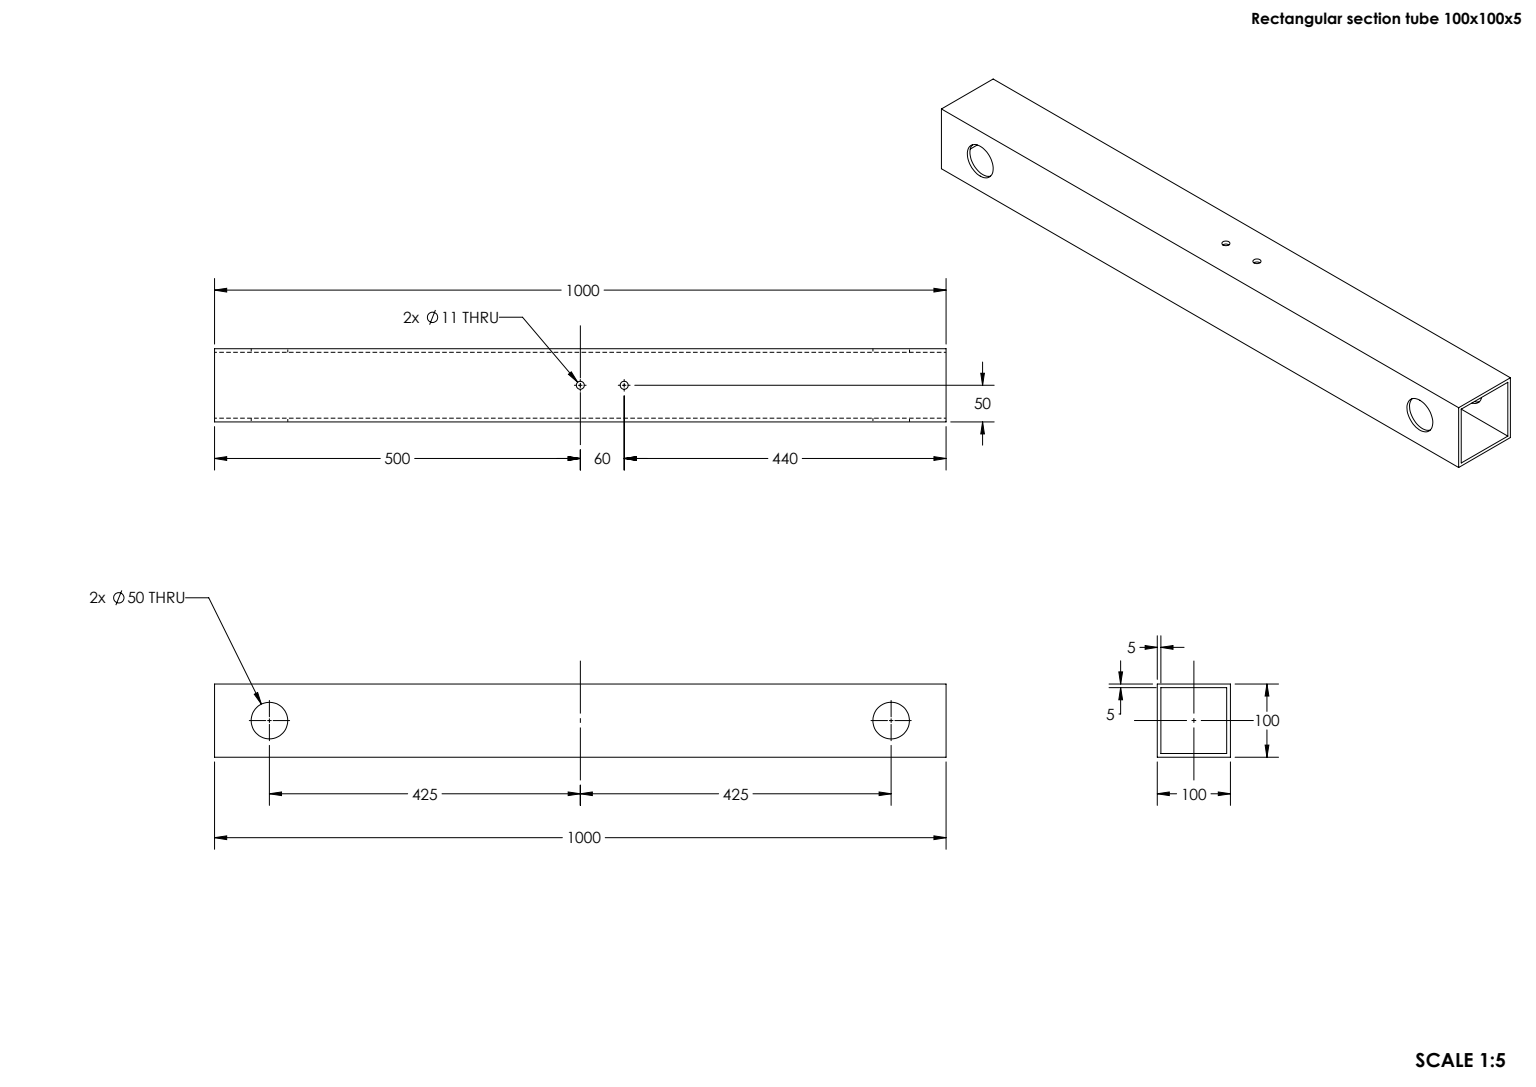
ISO-10303-21;
HEADER;
FILE_DESCRIPTION (('STEP AP214'),
    '1' );
FILE_NAME ('Rectangular section tube 100x100x5.step',
    '2026-10-24T15:53:57',
    ( '' ),
    ( '' ),
    'SwSTEP 2.0',
    'SolidWorks 2025',
    '' );
FILE_SCHEMA (( 'AUTOMOTIVE_DESIGN' ));
ENDSEC;

DATA;
#26=CYLINDRICAL_SURFACE ( 'NONE', #6690, 5.499999999999999112 ) ;
#33=ORIENTED_EDGE ( 'NONE', *, *, #2623, .F. ) ;
#38=VECTOR ( 'NONE', #5500, 1000.000000000000000 ) ;
#41=CARTESIAN_POINT ( 'NONE',  ( 44.99999999999992895, -425.0000000000000000, -3.122502256758253953E-15 ) ) ;
#48=EDGE_CURVE ( 'NONE', #6303, #1514, #1175, .T. ) ;
#52=ADVANCED_FACE ( 'NONE', ( #8577 ), #1878, .F. ) ;
#60=ORIENTED_EDGE ( 'NONE', *, *, #341, .F. ) ;
#66=CARTESIAN_POINT ( 'NONE',  ( 50.00000000000004263, 500.0000000000000000, -45.00000000000000711 ) ) ;
#95=FACE_BOUND ( 'NONE', #8531, .T. ) ;
#125=DIRECTION ( 'NONE',  ( 0.000000000000000000, -0.000000000000000000, 1.000000000000000000 ) ) ;
#127=EDGE_LOOP ( 'NONE', ( #5459, #6206, #3231, #7547 ) ) ;
#132=MANIFOLD_SOLID_BREP ( 'Cut-Extrude2', #7926 ) ;
#140=ORIENTED_EDGE ( 'NONE', *, *, #515, .T. ) ;
#141=VECTOR ( 'NONE', #1678, 1000.000000000000000 ) ;
#147=DIRECTION ( 'NONE',  ( 1.000000000000000000, 0.000000000000000000, 0.000000000000000000 ) ) ;
#163=DIRECTION ( 'NONE',  ( -1.000000000000000000, 0.000000000000000000, 6.938893903907228378E-17 ) ) ;
#164=AXIS2_PLACEMENT_3D ( 'NONE', #7493, #6114, #5025 ) ;
#179=CARTESIAN_POINT ( 'NONE',  ( 0.000000000000000000, 0.000000000000000000, -50.00000000000000000 ) ) ;
#181=VERTEX_POINT ( 'NONE', #3609 ) ;
#186=DIRECTION ( 'NONE',  ( 1.000000000000000000, 0.000000000000000000, 0.000000000000000000 ) ) ;
#201=CIRCLE ( 'NONE', #4665, 25.00000000000000711 ) ;
#206=CARTESIAN_POINT ( 'NONE',  ( -50.00000000000004263, 425.0000000000000000, 25.00000000000001066 ) ) ;
#219=EDGE_CURVE ( 'NONE', #4124, #477, #2955, .T. ) ;
#234=DIRECTION ( 'NONE',  ( 1.000000000000000000, 0.000000000000000000, 0.000000000000000000 ) ) ;
#248=ORIENTED_EDGE ( 'NONE', *, *, #4056, .T. ) ;
#263=FACE_OUTER_BOUND ( 'NONE', #2610, .T. ) ;
#264=ORIENTED_EDGE ( 'NONE', *, *, #6676, .F. ) ;
#267=DIRECTION ( 'NONE',  ( 1.000000000000000000, 0.000000000000000000, -0.000000000000000000 ) ) ;
#272=DIRECTION ( 'NONE',  ( -0.000000000000000000, -0.000000000000000000, 1.000000000000000000 ) ) ;
#317=DIRECTION ( 'NONE',  ( -1.000000000000000000, 0.000000000000000000, 0.000000000000000000 ) ) ;
#324=DIRECTION ( 'NONE',  ( 1.000000000000000000, 0.000000000000000000, 0.000000000000000000 ) ) ;
#330=CIRCLE ( 'NONE', #8396, 5.500000000000000000 ) ;
#341=EDGE_CURVE ( 'NONE', #5769, #3947, #5762, .T. ) ;
#360=CARTESIAN_POINT ( 'NONE',  ( 44.99999999999992895, -425.0000000000000000, 25.00000000000000355 ) ) ;
#378=CARTESIAN_POINT ( 'NONE',  ( 44.99999999999992895, 500.0000000000000000, 45.00000000000000711 ) ) ;
#383=AXIS2_PLACEMENT_3D ( 'NONE', #3939, #7208, #1372 ) ;
#384=CIRCLE ( 'NONE', #8575, 25.00000000000000711 ) ;
#389=DIRECTION ( 'NONE',  ( 0.000000000000000000, 0.000000000000000000, 1.000000000000000000 ) ) ;
#399=ORIENTED_EDGE ( 'NONE', *, *, #5241, .T. ) ;
#415=ORIENTED_EDGE ( 'NONE', *, *, #5873, .T. ) ;
#420=VECTOR ( 'NONE', #8328, 1000.000000000000000 ) ;
#423=DIRECTION ( 'NONE',  ( 0.000000000000000000, 0.000000000000000000, -1.000000000000000000 ) ) ;
#426=DIRECTION ( 'NONE',  ( -6.938893903907228378E-17, 0.000000000000000000, 1.000000000000000000 ) ) ;
#430=CARTESIAN_POINT ( 'NONE',  ( 5.500000000000000000, 0.000000000000000000, -50.00000000000000000 ) ) ;
#450=VERTEX_POINT ( 'NONE', #1353 ) ;
#476=DIRECTION ( 'NONE',  ( 1.000000000000000000, 0.000000000000000000, 0.000000000000000000 ) ) ;
#477=VERTEX_POINT ( 'NONE', #2037 ) ;
#512=EDGE_LOOP ( 'NONE', ( #2319, #8430 ) ) ;
#514=ORIENTED_EDGE ( 'NONE', *, *, #4418, .T. ) ;
#515=EDGE_CURVE ( 'NONE', #4124, #4726, #6274, .T. ) ;
#527=EDGE_LOOP ( 'NONE', ( #6886, #2691, #1406, #7538 ) ) ;
#534=ORIENTED_EDGE ( 'NONE', *, *, #219, .F. ) ;
#539=DIRECTION ( 'NONE',  ( -0.000000000000000000, -1.000000000000000000, -0.000000000000000000 ) ) ;
#542=AXIS2_PLACEMENT_3D ( 'NONE', #3104, #2449, #324 ) ;
#560=ORIENTED_EDGE ( 'NONE', *, *, #1216, .F. ) ;
#602=VECTOR ( 'NONE', #6763, 1000.000000000000000 ) ;
#615=DIRECTION ( 'NONE',  ( 1.000000000000000000, 0.000000000000000000, 0.000000000000000000 ) ) ;
#616=DIRECTION ( 'NONE',  ( -1.000000000000000000, 0.000000000000000000, 0.000000000000000000 ) ) ;
#633=PLANE ( 'NONE',  #383 ) ;
#636=CARTESIAN_POINT ( 'NONE',  ( -44.99999999999992895, 500.0000000000000000, -45.00000000000000711 ) ) ;
#643=EDGE_CURVE ( 'NONE', #5503, #8027, #3386, .T. ) ;
#666=ORIENTED_EDGE ( 'NONE', *, *, #745, .T. ) ;
#670=ORIENTED_EDGE ( 'NONE', *, *, #5204, .T. ) ;
#675=ORIENTED_EDGE ( 'NONE', *, *, #6201, .T. ) ;
#681=CARTESIAN_POINT ( 'NONE',  ( -5.499999999999999112, 60.00000000000000000, -50.00000000000000000 ) ) ;
#692=DIRECTION ( 'NONE',  ( 0.000000000000000000, -0.000000000000000000, 1.000000000000000000 ) ) ;
#695=ORIENTED_EDGE ( 'NONE', *, *, #4152, .T. ) ;
#696=ADVANCED_FACE ( 'NONE', ( #5758, #8388, #999 ), #4341, .F. ) ;
#708=EDGE_CURVE ( 'NONE', #8288, #1229, #2420, .T. ) ;
#711=DIRECTION ( 'NONE',  ( -1.000000000000000000, 0.000000000000000000, 6.938893903907228378E-17 ) ) ;
#715=ORIENTED_EDGE ( 'NONE', *, *, #8367, .T. ) ;
#719=DIRECTION ( 'NONE',  ( 6.938893903907228378E-17, 0.000000000000000000, -1.000000000000000000 ) ) ;
#720=CARTESIAN_POINT ( 'NONE',  ( 0.000000000000000000, 60.00000000000000000, -50.00000000000000000 ) ) ;
#724=VECTOR ( 'NONE', #6940, 1000.000000000000000 ) ;
#729=FACE_OUTER_BOUND ( 'NONE', #7779, .T. ) ;
#738=ORIENTED_EDGE ( 'NONE', *, *, #219, .T. ) ;
#745=EDGE_CURVE ( 'NONE', #3947, #6439, #5046, .T. ) ;
#747=FACE_OUTER_BOUND ( 'NONE', #3148, .T. ) ;
#748=VERTEX_POINT ( 'NONE', #4072 ) ;
#750=CIRCLE ( 'NONE', #2555, 5.500000000000000000 ) ;
#765=FACE_BOUND ( 'NONE', #1653, .T. ) ;
#766=EDGE_LOOP ( 'NONE', ( #2291, #6698, #7968, #2471 ) ) ;
#782=CARTESIAN_POINT ( 'NONE',  ( -50.00000000000004263, 425.0000000000000000, 25.00000000000001066 ) ) ;
#791=DIRECTION ( 'NONE',  ( -1.000000000000000000, 0.000000000000000000, -6.938893903907228378E-17 ) ) ;
#792=ORIENTED_EDGE ( 'NONE', *, *, #1046, .T. ) ;
#813=CARTESIAN_POINT ( 'NONE',  ( 0.000000000000000000, 0.000000000000000000, 45.00000000000000000 ) ) ;
#816=DIRECTION ( 'NONE',  ( 1.000000000000000000, -0.000000000000000000, -6.938893903907228378E-17 ) ) ;
#829=AXIS2_PLACEMENT_3D ( 'NONE', #8457, #1837, #1102 ) ;
#833=CARTESIAN_POINT ( 'NONE',  ( 5.500000000000000000, 0.000000000000000000, -45.00000000000000711 ) ) ;
#848=CARTESIAN_POINT ( 'NONE',  ( 0.000000000000000000, 0.000000000000000000, 50.00000000000000000 ) ) ;
#861=EDGE_LOOP ( 'NONE', ( #7328, #4385, #6462, #1916 ) ) ;
#864=DIRECTION ( 'NONE',  ( 1.000000000000000000, 0.000000000000000000, -6.938893903907228378E-17 ) ) ;
#876=VECTOR ( 'NONE', #539, 1000.000000000000000 ) ;
#880=VECTOR ( 'NONE', #1967, 1000.000000000000000 ) ;
#915=ORIENTED_EDGE ( 'NONE', *, *, #4440, .T. ) ;
#929=DIRECTION ( 'NONE',  ( 0.000000000000000000, -0.000000000000000000, 1.000000000000000000 ) ) ;
#940=ORIENTED_EDGE ( 'NONE', *, *, #515, .F. ) ;
#941=VECTOR ( 'NONE', #8021, 1000.000000000000000 ) ;
#950=DIRECTION ( 'NONE',  ( 1.000000000000000000, 0.000000000000000000, 0.000000000000000000 ) ) ;
#982=VERTEX_POINT ( 'NONE', #1520 ) ;
#988=VERTEX_POINT ( 'NONE', #6160 ) ;
#999=FACE_OUTER_BOUND ( 'NONE', #2827, .T. ) ;
#1010=EDGE_LOOP ( 'NONE', ( #4904, #534, #140, #1394 ) ) ;
#1011=ORIENTED_EDGE ( 'NONE', *, *, #5241, .F. ) ;
#1022=DIRECTION ( 'NONE',  ( -6.938893903907228378E-17, 0.000000000000000000, -1.000000000000000000 ) ) ;
#1041=CARTESIAN_POINT ( 'NONE',  ( 50.00000000000004263, -500.0000000000000000, -45.00000000000000711 ) ) ;
#1043=CARTESIAN_POINT ( 'NONE',  ( -5.499999999999999112, 60.00000000000000000, -45.00000000000000711 ) ) ;
#1046=EDGE_CURVE ( 'NONE', #7133, #5698, #2303, .T. ) ;
#1048=ORIENTED_EDGE ( 'NONE', *, *, #2437, .F. ) ;
#1091=VECTOR ( 'NONE', #8406, 1000.000000000000000 ) ;
#1102=DIRECTION ( 'NONE',  ( 0.000000000000000000, 0.000000000000000000, 1.000000000000000000 ) ) ;
#1106=ORIENTED_EDGE ( 'NONE', *, *, #8367, .F. ) ;
#1110=ADVANCED_FACE ( 'NONE', ( #7138 ), #5042, .F. ) ;
#1113=VECTOR ( 'NONE', #7329, 1000.000000000000000 ) ;
#1129=ORIENTED_EDGE ( 'NONE', *, *, #6644, .F. ) ;
#1146=DIRECTION ( 'NONE',  ( -0.000000000000000000, -0.000000000000000000, 1.000000000000000000 ) ) ;
#1153=AXIS2_PLACEMENT_3D ( 'NONE', #6835, #864, #4865 ) ;
#1166=DIRECTION ( 'NONE',  ( -0.000000000000000000, -1.000000000000000000, -0.000000000000000000 ) ) ;
#1175=LINE ( 'NONE', #6489, #2104 ) ;
#1203=DIRECTION ( 'NONE',  ( 1.000000000000000000, -0.000000000000000000, -6.938893903907228378E-17 ) ) ;
#1216=EDGE_CURVE ( 'NONE', #982, #5776, #7594, .T. ) ;
#1229=VERTEX_POINT ( 'NONE', #2040 ) ;
#1238=DIRECTION ( 'NONE',  ( -0.000000000000000000, -0.000000000000000000, 1.000000000000000000 ) ) ;
#1244=AXIS2_PLACEMENT_3D ( 'NONE', #8165, #2850, #7552 ) ;
#1313=DIRECTION ( 'NONE',  ( 0.000000000000000000, 0.000000000000000000, 1.000000000000000000 ) ) ;
#1320=DIRECTION ( 'NONE',  ( -6.938893903907228378E-17, 0.000000000000000000, -1.000000000000000000 ) ) ;
#1325=CARTESIAN_POINT ( 'NONE',  ( 50.00000000000004263, -500.0000000000000000, -50.00000000000000000 ) ) ;
#1332=CARTESIAN_POINT ( 'NONE',  ( -50.00000000000004263, -425.0000000000000000, 3.469446951953614189E-15 ) ) ;
#1340=DIRECTION ( 'NONE',  ( -0.000000000000000000, -1.000000000000000000, -0.000000000000000000 ) ) ;
#1342=EDGE_CURVE ( 'NONE', #450, #2950, #6967, .T. ) ;
#1344=AXIS2_PLACEMENT_3D ( 'NONE', #2202, #2124, #4896 ) ;
#1353=CARTESIAN_POINT ( 'NONE',  ( -50.00000000000004263, -425.0000000000000000, 25.00000000000001066 ) ) ;
#1372=DIRECTION ( 'NONE',  ( 1.000000000000000000, 0.000000000000000000, -0.000000000000000000 ) ) ;
#1394=ORIENTED_EDGE ( 'NONE', *, *, #8411, .T. ) ;
#1406=ORIENTED_EDGE ( 'NONE', *, *, #7155, .T. ) ;
#1423=( GEOMETRIC_REPRESENTATION_CONTEXT ( 3 ) GLOBAL_UNCERTAINTY_ASSIGNED_CONTEXT ( ( #7750 ) ) GLOBAL_UNIT_ASSIGNED_CONTEXT ( ( #7929, #7280, #4868 ) ) REPRESENTATION_CONTEXT ( 'NONE', 'WORKASPACE' ) );
#1442=DIRECTION ( 'NONE',  ( -0.000000000000000000, -0.000000000000000000, 1.000000000000000000 ) ) ;
#1448=AXIS2_PLACEMENT_3D ( 'NONE', #5599, #1778, #4966 ) ;
#1466=LINE ( 'NONE', #1940, #6330 ) ;
#1474=DIRECTION ( 'NONE',  ( 1.000000000000000000, 0.000000000000000000, -0.000000000000000000 ) ) ;
#1497=LINE ( 'NONE', #4154, #1568 ) ;
#1503=( NAMED_UNIT ( * ) SI_UNIT ( $, .STERADIAN. ) SOLID_ANGLE_UNIT ( ) );
#1510=CARTESIAN_POINT ( 'NONE',  ( -50.00000000000004263, -425.0000000000000000, 25.00000000000001066 ) ) ;
#1512=AXIS2_PLACEMENT_3D ( 'NONE', #66, #692, #1474 ) ;
#1514=VERTEX_POINT ( 'NONE', #6507 ) ;
#1520=CARTESIAN_POINT ( 'NONE',  ( 50.00000000000004263, 425.0000000000000000, 25.00000000000000355 ) ) ;
#1522=DIRECTION ( 'NONE',  ( 0.000000000000000000, 0.000000000000000000, 1.000000000000000000 ) ) ;
#1524=VERTEX_POINT ( 'NONE', #3199 ) ;
#1557=ORIENTED_EDGE ( 'NONE', *, *, #5889, .T. ) ;
#1568=VECTOR ( 'NONE', #6824, 1000.000000000000000 ) ;
#1573=ORIENTED_EDGE ( 'NONE', *, *, #4888, .F. ) ;
#1624=SHAPE_REPRESENTATION_RELATIONSHIP ( 'NONE' , 'NONE' ,  #4603, #2622 ) ;
#1639=VECTOR ( 'NONE', #4257, 1000.000000000000000 ) ;
#1653=EDGE_LOOP ( 'NONE', ( #738, #8439 ) ) ;
#1655=CARTESIAN_POINT ( 'NONE',  ( -44.99999999999992895, 425.0000000000000000, 3.122502256758253953E-15 ) ) ;
#1672=ADVANCED_FACE ( 'NONE', ( #765, #2549, #5205 ), #633, .F. ) ;
#1673=CARTESIAN_POINT ( 'NONE',  ( -50.00000000000004263, -500.0000000000000000, 50.00000000000000000 ) ) ;
#1678=DIRECTION ( 'NONE',  ( -0.000000000000000000, -1.000000000000000000, -0.000000000000000000 ) ) ;
#1693=ORIENTED_EDGE ( 'NONE', *, *, #5772, .T. ) ;
#1717=CARTESIAN_POINT ( 'NONE',  ( -50.00000000000004263, -425.0000000000000000, 3.469446951953614189E-15 ) ) ;
#1740=CARTESIAN_POINT ( 'NONE',  ( 0.000000000000000000, 0.000000000000000000, -50.00000000000000000 ) ) ;
#1742=VERTEX_POINT ( 'NONE', #6691 ) ;
#1745=CARTESIAN_POINT ( 'NONE',  ( -5.500000000000000000, 6.735557395310442023E-16, -50.00000000000000000 ) ) ;
#1747=EDGE_CURVE ( 'NONE', #3875, #4021, #7469, .T. ) ;
#1758=FACE_OUTER_BOUND ( 'NONE', #2934, .T. ) ;
#1759=EDGE_CURVE ( 'NONE', #4794, #4726, #3149, .T. ) ;
#1761=DIRECTION ( 'NONE',  ( 1.000000000000000000, -0.000000000000000000, -6.938893903907228378E-17 ) ) ;
#1778=DIRECTION ( 'NONE',  ( 1.000000000000000000, -0.000000000000000000, -6.938893903907228378E-17 ) ) ;
#1785=CARTESIAN_POINT ( 'NONE',  ( 50.00000000000004263, -425.0000000000000000, -25.00000000000001066 ) ) ;
#1790=AXIS2_PLACEMENT_3D ( 'NONE', #2424, #3035, #2511 ) ;
#1812=DIRECTION ( 'NONE',  ( 1.000000000000000000, 0.000000000000000000, -6.938893903907228378E-17 ) ) ;
#1826=EDGE_LOOP ( 'NONE', ( #2329, #3205, #514, #3584 ) ) ;
#1837=DIRECTION ( 'NONE',  ( -1.000000000000000000, 0.000000000000000000, 6.938893903907228378E-17 ) ) ;
#1845=ORIENTED_EDGE ( 'NONE', *, *, #6487, .T. ) ;
#1852=VECTOR ( 'NONE', #6126, 1000.000000000000000 ) ;
#1862=CARTESIAN_POINT ( 'NONE',  ( -50.00000000000004263, 500.0000000000000000, 50.00000000000000000 ) ) ;
#1872=EDGE_CURVE ( 'NONE', #988, #1514, #2766, .T. ) ;
#1878=CYLINDRICAL_SURFACE ( 'NONE', #4599, 25.00000000000000711 ) ;
#1889=ORIENTED_EDGE ( 'NONE', *, *, #6867, .T. ) ;
#1893=DIRECTION ( 'NONE',  ( -0.000000000000000000, -0.000000000000000000, 1.000000000000000000 ) ) ;
#1895=DIRECTION ( 'NONE',  ( 1.000000000000000000, 0.000000000000000000, -6.938893903907228378E-17 ) ) ;
#1901=ORIENTED_EDGE ( 'NONE', *, *, #3069, .T. ) ;
#1904=PLANE ( 'NONE',  #3247 ) ;
#1906=CARTESIAN_POINT ( 'NONE',  ( 50.00000000000004263, 425.0000000000000000, -25.00000000000001066 ) ) ;
#1916=ORIENTED_EDGE ( 'NONE', *, *, #4023, .T. ) ;
#1940=CARTESIAN_POINT ( 'NONE',  ( -50.00000000000004263, 425.0000000000000000, 25.00000000000001066 ) ) ;
#1944=VECTOR ( 'NONE', #1146, 1000.000000000000000 ) ;
#1954=FACE_BOUND ( 'NONE', #7294, .T. ) ;
#1967=DIRECTION ( 'NONE',  ( -1.000000000000000000, 0.000000000000000000, 0.000000000000000000 ) ) ;
#1976=CARTESIAN_POINT ( 'NONE',  ( 0.000000000000000000, -500.0000000000000000, 0.000000000000000000 ) ) ;
#1978=CARTESIAN_POINT ( 'NONE',  ( 5.500000000000000000, 0.000000000000000000, -50.00000000000000000 ) ) ;
#1984=AXIS2_PLACEMENT_3D ( 'NONE', #1976, #2679, #3369 ) ;
#1992=CARTESIAN_POINT ( 'NONE',  ( 0.000000000000000000, 500.0000000000000000, 0.000000000000000000 ) ) ;
#1993=EDGE_CURVE ( 'NONE', #4021, #3875, #4723, .T. ) ;
#2001=ORIENTED_EDGE ( 'NONE', *, *, #5652, .F. ) ;
#2004=EDGE_LOOP ( 'NONE', ( #670, #6292 ) ) ;
#2016=FACE_BOUND ( 'NONE', #7479, .T. ) ;
#2026=VECTOR ( 'NONE', #4909, 1000.000000000000000 ) ;
#2037=CARTESIAN_POINT ( 'NONE',  ( -5.499999999999999112, 60.00000000000000000, 45.00000000000000000 ) ) ;
#2040=CARTESIAN_POINT ( 'NONE',  ( -44.99999999999992895, -425.0000000000000000, -25.00000000000000355 ) ) ;
#2049=CARTESIAN_POINT ( 'NONE',  ( 50.00000000000004263, 500.0000000000000000, 45.00000000000000711 ) ) ;
#2053=CARTESIAN_POINT ( 'NONE',  ( -50.00000000000004263, 500.0000000000000000, 50.00000000000000000 ) ) ;
#2058=EDGE_CURVE ( 'NONE', #3844, #4655, #7635, .T. ) ;
#2066=EDGE_LOOP ( 'NONE', ( #5222, #5126, #6989, #2981 ) ) ;
#2071=ADVANCED_FACE ( 'NONE', ( #2984 ), #4376, .F. ) ;
#2082=CIRCLE ( 'NONE', #2342, 5.500000000000000000 ) ;
#2097=PLANE ( 'NONE',  #164 ) ;
#2099=CARTESIAN_POINT ( 'NONE',  ( -50.00000000000004263, 425.0000000000000000, -25.00000000000000355 ) ) ;
#2101=CIRCLE ( 'NONE', #6813, 25.00000000000000711 ) ;
#2103=CYLINDRICAL_SURFACE ( 'NONE', #3993, 5.499999999999999112 ) ;
#2104=VECTOR ( 'NONE', #616, 1000.000000000000000 ) ;
#2107=DIRECTION ( 'NONE',  ( 1.000000000000000000, 0.000000000000000000, -6.938893903907228378E-17 ) ) ;
#2124=DIRECTION ( 'NONE',  ( 0.000000000000000000, 0.000000000000000000, 1.000000000000000000 ) ) ;
#2135=CARTESIAN_POINT ( 'NONE',  ( 44.99999999999992895, 500.0000000000000000, 45.00000000000000711 ) ) ;
#2142=EDGE_LOOP ( 'NONE', ( #33, #1106, #248, #6182 ) ) ;
#2151=DIRECTION ( 'NONE',  ( 0.000000000000000000, 0.000000000000000000, 1.000000000000000000 ) ) ;
#2155=EDGE_CURVE ( 'NONE', #4565, #6245, #2101, .T. ) ;
#2167=VERTEX_POINT ( 'NONE', #2624 ) ;
#2189=ORIENTED_EDGE ( 'NONE', *, *, #2840, .T. ) ;
#2202=CARTESIAN_POINT ( 'NONE',  ( 0.000000000000000000, 60.00000000000000000, 50.00000000000000000 ) ) ;
#2222=DIRECTION ( 'NONE',  ( -6.938893903907228378E-17, 0.000000000000000000, -1.000000000000000000 ) ) ;
#2231=CYLINDRICAL_SURFACE ( 'NONE', #5281, 25.00000000000000711 ) ;
#2232=CIRCLE ( 'NONE', #7106, 25.00000000000000711 ) ;
#2242=ORIENTED_EDGE ( 'NONE', *, *, #3280, .F. ) ;
#2250=EDGE_CURVE ( 'NONE', #4067, #5769, #5139, .T. ) ;
#2251=CARTESIAN_POINT ( 'NONE',  ( 5.499999999999999112, 60.00000000000000000, -50.00000000000000000 ) ) ;
#2252=STYLED_ITEM('',(#8677),#132);
#2291=ORIENTED_EDGE ( 'NONE', *, *, #1747, .F. ) ;
#2303=LINE ( 'NONE', #2834, #38 ) ;
#2319=ORIENTED_EDGE ( 'NONE', *, *, #1993, .T. ) ;
#2329=ORIENTED_EDGE ( 'NONE', *, *, #8279, .F. ) ;
#2342=AXIS2_PLACEMENT_3D ( 'NONE', #3203, #8511, #5159 ) ;
#2356=CIRCLE ( 'NONE', #8206, 25.00000000000000711 ) ;
#2368=FACE_BOUND ( 'NONE', #7739, .T. ) ;
#2371=CYLINDRICAL_SURFACE ( 'NONE', #5767, 25.00000000000000711 ) ;
#2373=PRODUCT_DEFINITION_CONTEXT ( 'detailed design', #8581, 'design' ) ;
#2392=CIRCLE ( 'NONE', #6443, 25.00000000000000711 ) ;
#2393=VECTOR ( 'NONE', #719, 1000.000000000000000 ) ;
#2395=EDGE_CURVE ( 'NONE', #4021, #2167, #7762, .T. ) ;
#2398=DIRECTION ( 'NONE',  ( 6.938893903907228378E-17, 0.000000000000000000, 1.000000000000000000 ) ) ;
#2409=VECTOR ( 'NONE', #1320, 1000.000000000000000 ) ;
#2420=LINE ( 'NONE', #7082, #6730 ) ;
#2424=CARTESIAN_POINT ( 'NONE',  ( 0.000000000000000000, 60.00000000000000000, 45.00000000000000000 ) ) ;
#2437=EDGE_CURVE ( 'NONE', #3262, #4756, #8066, .T. ) ;
#2438=CYLINDRICAL_SURFACE ( 'NONE', #1448, 25.00000000000000711 ) ;
#2449=DIRECTION ( 'NONE',  ( 0.000000000000000000, 0.000000000000000000, 1.000000000000000000 ) ) ;
#2471=ORIENTED_EDGE ( 'NONE', *, *, #2395, .F. ) ;
#2489=CIRCLE ( 'NONE', #7501, 25.00000000000000711 ) ;
#2500=AXIS2_PLACEMENT_3D ( 'NONE', #848, #6172, #7420 ) ;
#2511=DIRECTION ( 'NONE',  ( 1.000000000000000000, 0.000000000000000000, 0.000000000000000000 ) ) ;
#2539=DIRECTION ( 'NONE',  ( 0.000000000000000000, 0.000000000000000000, 1.000000000000000000 ) ) ;
#2549=FACE_BOUND ( 'NONE', #6675, .T. ) ;
#2555=AXIS2_PLACEMENT_3D ( 'NONE', #4993, #389, #3036 ) ;
#2610=EDGE_LOOP ( 'NONE', ( #8303, #1573, #2915, #792 ) ) ;
#2611=CARTESIAN_POINT ( 'NONE',  ( 0.000000000000000000, 60.00000000000000000, -50.00000000000000000 ) ) ;
#2614=CIRCLE ( 'NONE', #8587, 25.00000000000000711 ) ;
#2616=CARTESIAN_POINT ( 'NONE',  ( -50.00000000000004263, -425.0000000000000000, 3.469446951953614189E-15 ) ) ;
#2622=ADVANCED_BREP_SHAPE_REPRESENTATION ( '', ( #132, #7563 ), #3529 ) ;
#2623=EDGE_CURVE ( 'NONE', #6630, #4756, #8454, .T. ) ;
#2624=CARTESIAN_POINT ( 'NONE',  ( 5.499999999999999112, 60.00000000000000000, -45.00000000000000711 ) ) ;
#2632=ORIENTED_EDGE ( 'NONE', *, *, #4023, .F. ) ;
#2633=CARTESIAN_POINT ( 'NONE',  ( 5.500000000000000000, 0.000000000000000000, 50.00000000000000000 ) ) ;
#2640=DIRECTION ( 'NONE',  ( -0.000000000000000000, -0.000000000000000000, 1.000000000000000000 ) ) ;
#2645=CARTESIAN_POINT ( 'NONE',  ( 50.00000000000004263, -500.0000000000000000, 50.00000000000000000 ) ) ;
#2653=EDGE_CURVE ( 'NONE', #7133, #2971, #7113, .T. ) ;
#2670=SHAPE_DEFINITION_REPRESENTATION ( #4043, #4603 ) ;
#2676=ORIENTED_EDGE ( 'NONE', *, *, #6819, .T. ) ;
#2679=DIRECTION ( 'NONE',  ( 0.000000000000000000, 1.000000000000000000, 0.000000000000000000 ) ) ;
#2691=ORIENTED_EDGE ( 'NONE', *, *, #2623, .T. ) ;
#2710=CARTESIAN_POINT ( 'NONE',  ( 50.00000000000004263, 425.0000000000000000, -3.469446951953614189E-15 ) ) ;
#2728=PRODUCT ( 'Rectangular section tube 100x100x5', 'Rectangular section tube 100x100x5', '', ( #3877 ) ) ;
#2730=CARTESIAN_POINT ( 'NONE',  ( -5.500000000000000000, 6.735557395310442023E-16, 45.00000000000000000 ) ) ;
#2742=LINE ( 'NONE', #6704, #4720 ) ;
#2744=LINE ( 'NONE', #782, #7445 ) ;
#2745=ORIENTED_EDGE ( 'NONE', *, *, #7556, .T. ) ;
#2749=FACE_OUTER_BOUND ( 'NONE', #3005, .T. ) ;
#2755=ORIENTED_EDGE ( 'NONE', *, *, #6644, .T. ) ;
#2766=LINE ( 'NONE', #8128, #6235 ) ;
#2773=ORIENTED_EDGE ( 'NONE', *, *, #3587, .T. ) ;
#2787=DIRECTION ( 'NONE',  ( 0.000000000000000000, -0.000000000000000000, 1.000000000000000000 ) ) ;
#2794=DIRECTION ( 'NONE',  ( 1.000000000000000000, 0.000000000000000000, -0.000000000000000000 ) ) ;
#2827=EDGE_LOOP ( 'NONE', ( #695, #6875, #6894, #4818 ) ) ;
#2833=DIRECTION ( 'NONE',  ( 0.000000000000000000, 0.000000000000000000, 1.000000000000000000 ) ) ;
#2834=CARTESIAN_POINT ( 'NONE',  ( 50.00000000000004263, 500.0000000000000000, 50.00000000000000000 ) ) ;
#2839=EDGE_LOOP ( 'NONE', ( #6572, #7525, #6505, #4873 ) ) ;
#2840=EDGE_CURVE ( 'NONE', #7133, #6524, #5682, .T. ) ;
#2850=DIRECTION ( 'NONE',  ( 1.000000000000000000, 0.000000000000000000, -6.938893903907228378E-17 ) ) ;
#2860=EDGE_LOOP ( 'NONE', ( #7495, #6369, #7792, #8428 ) ) ;
#2876=ORIENTED_EDGE ( 'NONE', *, *, #6819, .F. ) ;
#2907=ORIENTED_EDGE ( 'NONE', *, *, #4501, .F. ) ;
#2913=AXIS2_PLACEMENT_3D ( 'NONE', #1332, #1895, #3941 ) ;
#2915=ORIENTED_EDGE ( 'NONE', *, *, #2653, .F. ) ;
#2924=EDGE_CURVE ( 'NONE', #1524, #4837, #2952, .T. ) ;
#2927=DIRECTION ( 'NONE',  ( -1.000000000000000000, 0.000000000000000000, 6.938893903907228378E-17 ) ) ;
#2934=EDGE_LOOP ( 'NONE', ( #5981, #8102, #1693, #399 ) ) ;
#2941=MECHANICAL_DESIGN_GEOMETRIC_PRESENTATION_REPRESENTATION('',(#2252),#1423);
#2950=VERTEX_POINT ( 'NONE', #7257 ) ;
#2952=LINE ( 'NONE', #5635, #141 ) ;
#2955=CIRCLE ( 'NONE', #6995, 5.499999999999999112 ) ;
#2971=VERTEX_POINT ( 'NONE', #7438 ) ;
#2981=ORIENTED_EDGE ( 'NONE', *, *, #4888, .T. ) ;
#2984=FACE_OUTER_BOUND ( 'NONE', #4206, .T. ) ;
#2985=ORIENTED_EDGE ( 'NONE', *, *, #2395, .T. ) ;
#3005=EDGE_LOOP ( 'NONE', ( #3658, #8012, #2985, #5669 ) ) ;
#3014=CARTESIAN_POINT ( 'NONE',  ( 50.00000000000004263, 500.0000000000000000, 50.00000000000000000 ) ) ;
#3026=ORIENTED_EDGE ( 'NONE', *, *, #8231, .F. ) ;
#3027=FACE_OUTER_BOUND ( 'NONE', #861, .T. ) ;
#3035=DIRECTION ( 'NONE',  ( 0.000000000000000000, -0.000000000000000000, 1.000000000000000000 ) ) ;
#3036=DIRECTION ( 'NONE',  ( 1.000000000000000000, 0.000000000000000000, 0.000000000000000000 ) ) ;
#3069=EDGE_CURVE ( 'NONE', #3768, #748, #4983, .T. ) ;
#3104=CARTESIAN_POINT ( 'NONE',  ( 0.000000000000000000, 60.00000000000000000, -50.00000000000000000 ) ) ;
#3119=PRODUCT_DEFINITION_FORMATION_WITH_SPECIFIED_SOURCE ( 'ANY', '', #2728, .NOT_KNOWN. ) ;
#3124=EDGE_LOOP ( 'NONE', ( #5831, #1557, #5683, #7930 ) ) ;
#3148=EDGE_LOOP ( 'NONE', ( #4973, #8440, #2189, #2676 ) ) ;
#3149=CIRCLE ( 'NONE', #1344, 5.499999999999999112 ) ;
#3199=CARTESIAN_POINT ( 'NONE',  ( -50.00000000000004263, 500.0000000000000000, -50.00000000000000000 ) ) ;
#3203=CARTESIAN_POINT ( 'NONE',  ( 0.000000000000000000, 0.000000000000000000, -45.00000000000000711 ) ) ;
#3205=ORIENTED_EDGE ( 'NONE', *, *, #3280, .T. ) ;
#3225=ADVANCED_FACE ( 'NONE', ( #4223 ), #8183, .F. ) ;
#3231=ORIENTED_EDGE ( 'NONE', *, *, #6487, .F. ) ;
#3244=ADVANCED_FACE ( 'NONE', ( #8054, #2368, #3027 ), #2097, .T. ) ;
#3245=CYLINDRICAL_SURFACE ( 'NONE', #4195, 5.500000000000000000 ) ;
#3247=AXIS2_PLACEMENT_3D ( 'NONE', #1992, #4560, #3387 ) ;
#3258=ORIENTED_EDGE ( 'NONE', *, *, #6503, .F. ) ;
#3262=VERTEX_POINT ( 'NONE', #833 ) ;
#3267=DIRECTION ( 'NONE',  ( -0.000000000000000000, -0.000000000000000000, 1.000000000000000000 ) ) ;
#3274=ORIENTED_EDGE ( 'NONE', *, *, #4440, .F. ) ;
#3280=EDGE_CURVE ( 'NONE', #4655, #3844, #2392, .T. ) ;
#3282=FACE_OUTER_BOUND ( 'NONE', #2142, .T. ) ;
#3284=CARTESIAN_POINT ( 'NONE',  ( 50.00000000000004263, -425.0000000000000000, 25.00000000000000355 ) ) ;
#3290=LINE ( 'NONE', #2645, #5576 ) ;
#3310=CARTESIAN_POINT ( 'NONE',  ( 50.00000000000004263, 500.0000000000000000, 50.00000000000000000 ) ) ;
#3311=DIRECTION ( 'NONE',  ( 0.000000000000000000, 0.000000000000000000, -1.000000000000000000 ) ) ;
#3320=CARTESIAN_POINT ( 'NONE',  ( 0.000000000000000000, 0.000000000000000000, -45.00000000000000711 ) ) ;
#3350=EDGE_LOOP ( 'NONE', ( #3026, #3682, #5381, #264 ) ) ;
#3369=DIRECTION ( 'NONE',  ( 0.000000000000000000, -0.000000000000000000, 1.000000000000000000 ) ) ;
#3386=CIRCLE ( 'NONE', #1153, 25.00000000000000711 ) ;
#3387=DIRECTION ( 'NONE',  ( 0.000000000000000000, -0.000000000000000000, 1.000000000000000000 ) ) ;
#3400=CARTESIAN_POINT ( 'NONE',  ( -50.00000000000004263, -500.0000000000000000, 50.00000000000000000 ) ) ;
#3428=DIRECTION ( 'NONE',  ( 0.000000000000000000, 0.000000000000000000, -1.000000000000000000 ) ) ;
#3440=DIRECTION ( 'NONE',  ( 1.000000000000000000, -0.000000000000000000, -6.938893903907228378E-17 ) ) ;
#3448=CARTESIAN_POINT ( 'NONE',  ( 44.99999999999992895, -425.0000000000000000, -3.122502256758253953E-15 ) ) ;
#3452=ORIENTED_EDGE ( 'NONE', *, *, #2653, .T. ) ;
#3458=CARTESIAN_POINT ( 'NONE',  ( -5.499999999999999112, 60.00000000000000000, -50.00000000000000000 ) ) ;
#3496=CARTESIAN_POINT ( 'NONE',  ( 44.99999999999992895, 425.0000000000000000, 25.00000000000000355 ) ) ;
#3497=ADVANCED_FACE ( 'NONE', ( #4725, #4685 ), #5291, .F. ) ;
#3499=DIRECTION ( 'NONE',  ( 1.000000000000000000, -0.000000000000000000, -6.938893903907228378E-17 ) ) ;
#3502=ORIENTED_EDGE ( 'NONE', *, *, #745, .F. ) ;
#3512=DIRECTION ( 'NONE',  ( 1.000000000000000000, 0.000000000000000000, 0.000000000000000000 ) ) ;
#3526=AXIS2_PLACEMENT_3D ( 'NONE', #6869, #3554, #234 ) ;
#3529=( GEOMETRIC_REPRESENTATION_CONTEXT ( 3 ) GLOBAL_UNCERTAINTY_ASSIGNED_CONTEXT ( ( #4657 ) ) GLOBAL_UNIT_ASSIGNED_CONTEXT ( ( #5392, #4735, #1503 ) ) REPRESENTATION_CONTEXT ( 'NONE', 'WORKASPACE' ) );
#3532=CARTESIAN_POINT ( 'NONE',  ( 5.500000000000000000, 0.000000000000000000, 45.00000000000000000 ) ) ;
#3548=VERTEX_POINT ( 'NONE', #1325 ) ;
#3554=DIRECTION ( 'NONE',  ( 0.000000000000000000, 0.000000000000000000, 1.000000000000000000 ) ) ;
#3579=LINE ( 'NONE', #4227, #8076 ) ;
#3584=ORIENTED_EDGE ( 'NONE', *, *, #6503, .T. ) ;
#3587=EDGE_CURVE ( 'NONE', #2971, #1524, #8537, .T. ) ;
#3588=CARTESIAN_POINT ( 'NONE',  ( -50.00000000000004263, -425.0000000000000000, 3.469446951953614189E-15 ) ) ;
#3593=CARTESIAN_POINT ( 'NONE',  ( 50.00000000000004263, 500.0000000000000000, -50.00000000000000000 ) ) ;
#3596=CARTESIAN_POINT ( 'NONE',  ( -50.00000000000004263, 425.0000000000000000, 3.469446951953614189E-15 ) ) ;
#3603=ORIENTED_EDGE ( 'NONE', *, *, #6676, .T. ) ;
#3604=EDGE_LOOP ( 'NONE', ( #6045, #6521, #3691, #666 ) ) ;
#3609=CARTESIAN_POINT ( 'NONE',  ( -50.00000000000004263, 425.0000000000000000, -25.00000000000000355 ) ) ;
#3639=ORIENTED_EDGE ( 'NONE', *, *, #5889, .F. ) ;
#3652=CARTESIAN_POINT ( 'NONE',  ( -44.99999999999992895, 500.0000000000000000, 50.00000000000000000 ) ) ;
#3658=ORIENTED_EDGE ( 'NONE', *, *, #5491, .F. ) ;
#3682=ORIENTED_EDGE ( 'NONE', *, *, #8558, .T. ) ;
#3691=ORIENTED_EDGE ( 'NONE', *, *, #341, .T. ) ;
#3724=DIRECTION ( 'NONE',  ( 1.000000000000000000, 0.000000000000000000, 0.000000000000000000 ) ) ;
#3736=CARTESIAN_POINT ( 'NONE',  ( -44.99999999999992895, -425.0000000000000000, 3.122502256758253953E-15 ) ) ;
#3755=CIRCLE ( 'NONE', #1244, 25.00000000000000711 ) ;
#3760=CARTESIAN_POINT ( 'NONE',  ( 44.99999999999992895, -500.0000000000000000, 50.00000000000000000 ) ) ;
#3768=VERTEX_POINT ( 'NONE', #2135 ) ;
#3802=AXIS2_PLACEMENT_3D ( 'NONE', #5253, #2640, #4123 ) ;
#3810=ORIENTED_EDGE ( 'NONE', *, *, #4663, .T. ) ;
#3814=CARTESIAN_POINT ( 'NONE',  ( -44.99999999999992895, -425.0000000000000000, 3.122502256758253953E-15 ) ) ;
#3844=VERTEX_POINT ( 'NONE', #8465 ) ;
#3858=DIRECTION ( 'NONE',  ( 0.000000000000000000, 0.000000000000000000, -1.000000000000000000 ) ) ;
#3860=PLANE ( 'NONE',  #7602 ) ;
#3861=DIRECTION ( 'NONE',  ( 0.000000000000000000, 0.000000000000000000, -1.000000000000000000 ) ) ;
#3870=CARTESIAN_POINT ( 'NONE',  ( -5.500000000000000000, 6.735557395310442023E-16, -45.00000000000000711 ) ) ;
#3875=VERTEX_POINT ( 'NONE', #7123 ) ;
#3877=PRODUCT_CONTEXT ( 'NONE', #4138, 'mechanical' ) ;
#3908=EDGE_LOOP ( 'NONE', ( #4614, #6053 ) ) ;
#3920=ADVANCED_FACE ( 'NONE', ( #1758 ), #2371, .F. ) ;
#3924=LINE ( 'NONE', #7287, #2409 ) ;
#3939=CARTESIAN_POINT ( 'NONE',  ( 50.00000000000004263, 500.0000000000000000, 45.00000000000000711 ) ) ;
#3941=DIRECTION ( 'NONE',  ( 0.000000000000000000, 0.000000000000000000, -1.000000000000000000 ) ) ;
#3947=VERTEX_POINT ( 'NONE', #2633 ) ;
#3951=FACE_BOUND ( 'NONE', #8129, .T. ) ;
#3954=DIRECTION ( 'NONE',  ( -6.938893903907228378E-17, 0.000000000000000000, 1.000000000000000000 ) ) ;
#3966=LINE ( 'NONE', #3400, #602 ) ;
#3967=VECTOR ( 'NONE', #4467, 1000.000000000000000 ) ;
#3971=DIRECTION ( 'NONE',  ( 1.000000000000000000, -0.000000000000000000, -6.938893903907228378E-17 ) ) ;
#3993=AXIS2_PLACEMENT_3D ( 'NONE', #4299, #1442, #4097 ) ;
#3994=EDGE_CURVE ( 'NONE', #6524, #1524, #6689, .T. ) ;
#4021=VERTEX_POINT ( 'NONE', #7334 ) ;
#4023=EDGE_CURVE ( 'NONE', #6303, #6735, #6055, .T. ) ;
#4043=PRODUCT_DEFINITION_SHAPE ( 'NONE', 'NONE',  #7892 ) ;
#4052=FACE_OUTER_BOUND ( 'NONE', #5336, .T. ) ;
#4056=EDGE_CURVE ( 'NONE', #1742, #3262, #7946, .T. ) ;
#4067=VERTEX_POINT ( 'NONE', #2730 ) ;
#4072=CARTESIAN_POINT ( 'NONE',  ( 44.99999999999992895, -500.0000000000000000, 45.00000000000000711 ) ) ;
#4087=AXIS2_PLACEMENT_3D ( 'NONE', #6626, #2787, #5987 ) ;
#4090=FACE_BOUND ( 'NONE', #6071, .T. ) ;
#4096=DIRECTION ( 'NONE',  ( -0.000000000000000000, -0.000000000000000000, 1.000000000000000000 ) ) ;
#4097=DIRECTION ( 'NONE',  ( 1.000000000000000000, 0.000000000000000000, 0.000000000000000000 ) ) ;
#4123=DIRECTION ( 'NONE',  ( 1.000000000000000000, 0.000000000000000000, 0.000000000000000000 ) ) ;
#4124=VERTEX_POINT ( 'NONE', #7555 ) ;
#4138=APPLICATION_CONTEXT ( 'automotive_design' ) ;
#4152=EDGE_CURVE ( 'NONE', #7562, #6221, #1497, .T. ) ;
#4154=CARTESIAN_POINT ( 'NONE',  ( -44.99999999999992895, -500.0000000000000000, 50.00000000000000000 ) ) ;
#4168=AXIS2_PLACEMENT_3D ( 'NONE', #3593, #5602, #267 ) ;
#4175=CARTESIAN_POINT ( 'NONE',  ( 44.99999999999992895, 425.0000000000000000, -3.122502256758253953E-15 ) ) ;
#4195=AXIS2_PLACEMENT_3D ( 'NONE', #4731, #1893, #6509 ) ;
#4202=AXIS2_PLACEMENT_3D ( 'NONE', #7454, #6241, #8342 ) ;
#4203=CARTESIAN_POINT ( 'NONE',  ( 0.000000000000000000, 0.000000000000000000, 0.000000000000000000 ) ) ;
#4206=EDGE_LOOP ( 'NONE', ( #8031, #1889, #6575, #60 ) ) ;
#4221=AXIS2_PLACEMENT_3D ( 'NONE', #2710, #2107, #1313 ) ;
#4223=FACE_OUTER_BOUND ( 'NONE', #527, .T. ) ;
#4226=AXIS2_PLACEMENT_3D ( 'NONE', #8473, #6438, #476 ) ;
#4227=CARTESIAN_POINT ( 'NONE',  ( -50.00000000000004263, -425.0000000000000000, -25.00000000000000355 ) ) ;
#4237=AXIS2_PLACEMENT_3D ( 'NONE', #813, #6144, #147 ) ;
#4240=PLANE ( 'NONE',  #4168 ) ;
#4244=DIRECTION ( 'NONE',  ( 1.000000000000000000, 0.000000000000000000, -6.938893903907228378E-17 ) ) ;
#4245=ORIENTED_EDGE ( 'NONE', *, *, #5145, .T. ) ;
#4257=DIRECTION ( 'NONE',  ( -0.000000000000000000, -0.000000000000000000, 1.000000000000000000 ) ) ;
#4278=FACE_OUTER_BOUND ( 'NONE', #2066, .T. ) ;
#4298=CIRCLE ( 'NONE', #1790, 5.499999999999999112 ) ;
#4299=CARTESIAN_POINT ( 'NONE',  ( 0.000000000000000000, 60.00000000000000000, -50.00000000000000000 ) ) ;
#4341=PLANE ( 'NONE',  #7009 ) ;
#4376=CYLINDRICAL_SURFACE ( 'NONE', #8459, 5.500000000000000000 ) ;
#4385=ORIENTED_EDGE ( 'NONE', *, *, #3069, .F. ) ;
#4388=EDGE_CURVE ( 'NONE', #5867, #4837, #3966, .T. ) ;
#4399=DIRECTION ( 'NONE',  ( 0.000000000000000000, 0.000000000000000000, 1.000000000000000000 ) ) ;
#4406=FACE_OUTER_BOUND ( 'NONE', #3604, .T. ) ;
#4410=ADVANCED_FACE ( 'NONE', ( #2749 ), #26, .F. ) ;
#4418=EDGE_CURVE ( 'NONE', #3844, #5776, #5364, .T. ) ;
#4427=EDGE_CURVE ( 'NONE', #2167, #7175, #8528, .T. ) ;
#4436=CARTESIAN_POINT ( 'NONE',  ( -50.00000000000004263, 425.0000000000000000, -25.00000000000000355 ) ) ;
#4440=EDGE_CURVE ( 'NONE', #3768, #988, #8019, .T. ) ;
#4454=ADVANCED_FACE ( 'NONE', ( #4052, #3951 ), #1904, .T. ) ;
#4460=ORIENTED_EDGE ( 'NONE', *, *, #3994, .F. ) ;
#4467=DIRECTION ( 'NONE',  ( 1.000000000000000000, -0.000000000000000000, -6.938893903907228378E-17 ) ) ;
#4501=EDGE_CURVE ( 'NONE', #5698, #3548, #3924, .T. ) ;
#4511=LINE ( 'NONE', #681, #7588 ) ;
#4524=LINE ( 'NONE', #4436, #1091 ) ;
#4548=CARTESIAN_POINT ( 'NONE',  ( 44.99999999999992895, 500.0000000000000000, -45.00000000000000711 ) ) ;
#4560=DIRECTION ( 'NONE',  ( 0.000000000000000000, 1.000000000000000000, 0.000000000000000000 ) ) ;
#4565=VERTEX_POINT ( 'NONE', #6212 ) ;
#4588=ADVANCED_FACE ( 'NONE', ( #4807 ), #7463, .F. ) ;
#4593=AXIS2_PLACEMENT_3D ( 'NONE', #5850, #8477, #3858 ) ;
#4599=AXIS2_PLACEMENT_3D ( 'NONE', #2616, #3971, #3311 ) ;
#4601=DIRECTION ( 'NONE',  ( 1.000000000000000000, 0.000000000000000000, 0.000000000000000000 ) ) ;
#4603=SHAPE_REPRESENTATION ( 'Rectangular section tube 100x100x5', ( #7563 ), #3529 ) ;
#4614=ORIENTED_EDGE ( 'NONE', *, *, #2155, .F. ) ;
#4616=ORIENTED_EDGE ( 'NONE', *, *, #4388, .F. ) ;
#4624=FACE_BOUND ( 'NONE', #8145, .T. ) ;
#4629=EDGE_CURVE ( 'NONE', #477, #4794, #6775, .T. ) ;
#4647=DIRECTION ( 'NONE',  ( -0.000000000000000000, -0.000000000000000000, 1.000000000000000000 ) ) ;
#4655=VERTEX_POINT ( 'NONE', #3496 ) ;
#4657=UNCERTAINTY_MEASURE_WITH_UNIT (LENGTH_MEASURE( 1.000000000000000082E-05 ), #5392, 'distance_accuracy_value', 'NONE');
#4663=EDGE_CURVE ( 'NONE', #6630, #1742, #330, .T. ) ;
#4665=AXIS2_PLACEMENT_3D ( 'NONE', #7449, #6800, #5492 ) ;
#4685=FACE_BOUND ( 'NONE', #3124, .T. ) ;
#4699=LINE ( 'NONE', #7345, #8301 ) ;
#4711=FACE_OUTER_BOUND ( 'NONE', #1010, .T. ) ;
#4720=VECTOR ( 'NONE', #5943, 1000.000000000000000 ) ;
#4723=CIRCLE ( 'NONE', #542, 5.499999999999999112 ) ;
#4725=FACE_OUTER_BOUND ( 'NONE', #7797, .T. ) ;
#4726=VERTEX_POINT ( 'NONE', #5781 ) ;
#4728=ADVANCED_FACE ( 'NONE', ( #8412 ), #2438, .F. ) ;
#4731=CARTESIAN_POINT ( 'NONE',  ( 0.000000000000000000, 0.000000000000000000, -50.00000000000000000 ) ) ;
#4735=( NAMED_UNIT ( * ) PLANE_ANGLE_UNIT ( ) SI_UNIT ( $, .RADIAN. ) );
#4749=FACE_OUTER_BOUND ( 'NONE', #6200, .T. ) ;
#4756=VERTEX_POINT ( 'NONE', #3870 ) ;
#4777=CIRCLE ( 'NONE', #7135, 25.00000000000000711 ) ;
#4782=CYLINDRICAL_SURFACE ( 'NONE', #7981, 25.00000000000000711 ) ;
#4794=VERTEX_POINT ( 'NONE', #7318 ) ;
#4805=VECTOR ( 'NONE', #8056, 1000.000000000000000 ) ;
#4807=FACE_OUTER_BOUND ( 'NONE', #2839, .T. ) ;
#4818=ORIENTED_EDGE ( 'NONE', *, *, #5652, .T. ) ;
#4835=ORIENTED_EDGE ( 'NONE', *, *, #48, .F. ) ;
#4837=VERTEX_POINT ( 'NONE', #5181 ) ;
#4863=CARTESIAN_POINT ( 'NONE',  ( 50.00000000000004263, -500.0000000000000000, 50.00000000000000000 ) ) ;
#4865=DIRECTION ( 'NONE',  ( 0.000000000000000000, 0.000000000000000000, -1.000000000000000000 ) ) ;
#4868=( NAMED_UNIT ( * ) SI_UNIT ( $, .STERADIAN. ) SOLID_ANGLE_UNIT ( ) );
#4873=ORIENTED_EDGE ( 'NONE', *, *, #5772, .F. ) ;
#4882=ORIENTED_EDGE ( 'NONE', *, *, #5147, .T. ) ;
#4885=DIRECTION ( 'NONE',  ( 1.000000000000000000, -0.000000000000000000, -6.938893903907228378E-17 ) ) ;
#4886=ORIENTED_EDGE ( 'NONE', *, *, #7969, .F. ) ;
#4888=EDGE_CURVE ( 'NONE', #2971, #3548, #4948, .T. ) ;
#4896=DIRECTION ( 'NONE',  ( 1.000000000000000000, 0.000000000000000000, 0.000000000000000000 ) ) ;
#4904=ORIENTED_EDGE ( 'NONE', *, *, #4629, .F. ) ;
#4909=DIRECTION ( 'NONE',  ( 1.000000000000000000, -0.000000000000000000, -6.938893903907228378E-17 ) ) ;
#4925=ADVANCED_FACE ( 'NONE', ( #4711 ), #2103, .F. ) ;
#4929=CARTESIAN_POINT ( 'NONE',  ( 0.000000000000000000, 0.000000000000000000, 45.00000000000000000 ) ) ;
#4941=ORIENTED_EDGE ( 'NONE', *, *, #4629, .T. ) ;
#4947=AXIS2_PLACEMENT_3D ( 'NONE', #7179, #7704, #4399 ) ;
#4948=LINE ( 'NONE', #6714, #941 ) ;
#4954=LINE ( 'NONE', #7774, #3967 ) ;
#4963=EDGE_LOOP ( 'NONE', ( #5124, #4941, #6929, #940 ) ) ;
#4966=DIRECTION ( 'NONE',  ( 0.000000000000000000, 0.000000000000000000, -1.000000000000000000 ) ) ;
#4973=ORIENTED_EDGE ( 'NONE', *, *, #5145, .F. ) ;
#4977=CARTESIAN_POINT ( 'NONE',  ( 0.000000000000000000, 0.000000000000000000, -50.00000000000000000 ) ) ;
#4982=EDGE_CURVE ( 'NONE', #6245, #4565, #384, .T. ) ;
#4983=LINE ( 'NONE', #378, #6564 ) ;
#4993=CARTESIAN_POINT ( 'NONE',  ( 0.000000000000000000, 0.000000000000000000, -50.00000000000000000 ) ) ;
#4994=ORIENTED_EDGE ( 'NONE', *, *, #4388, .T. ) ;
#5024=ORIENTED_EDGE ( 'NONE', *, *, #6539, .F. ) ;
#5025=DIRECTION ( 'NONE',  ( 6.938893903907228378E-17, 0.000000000000000000, 1.000000000000000000 ) ) ;
#5034=DIRECTION ( 'NONE',  ( -0.000000000000000000, -0.000000000000000000, 1.000000000000000000 ) ) ;
#5042=CYLINDRICAL_SURFACE ( 'NONE', #6471, 25.00000000000000711 ) ;
#5046=CIRCLE ( 'NONE', #3526, 5.500000000000000000 ) ;
#5072=DIRECTION ( 'NONE',  ( -1.000000000000000000, 0.000000000000000000, -6.938893903907228378E-17 ) ) ;
#5111=LINE ( 'NONE', #1041, #8223 ) ;
#5120=ADVANCED_FACE ( 'NONE', ( #8516 ), #7909, .F. ) ;
#5124=ORIENTED_EDGE ( 'NONE', *, *, #7145, .F. ) ;
#5126=ORIENTED_EDGE ( 'NONE', *, *, #2924, .F. ) ;
#5130=AXIS2_PLACEMENT_3D ( 'NONE', #3596, #4244, #7510 ) ;
#5136=AXIS2_PLACEMENT_3D ( 'NONE', #5466, #929, #6255 ) ;
#5138=LINE ( 'NONE', #3760, #6411 ) ;
#5139=CIRCLE ( 'NONE', #8485, 5.500000000000000000 ) ;
#5145=EDGE_CURVE ( 'NONE', #5698, #5867, #3290, .T. ) ;
#5147=EDGE_CURVE ( 'NONE', #5920, #5838, #2356, .T. ) ;
#5159=DIRECTION ( 'NONE',  ( 1.000000000000000000, 0.000000000000000000, 0.000000000000000000 ) ) ;
#5166=ADVANCED_FACE ( 'NONE', ( #5606 ), #6994, .F. ) ;
#5181=CARTESIAN_POINT ( 'NONE',  ( -50.00000000000004263, -500.0000000000000000, -50.00000000000000000 ) ) ;
#5183=AXIS2_PLACEMENT_3D ( 'NONE', #3310, #125, #2794 ) ;
#5186=EDGE_LOOP ( 'NONE', ( #6163, #7686, #6526, #5941 ) ) ;
#5199=ORIENTED_EDGE ( 'NONE', *, *, #8411, .F. ) ;
#5204=EDGE_CURVE ( 'NONE', #181, #8316, #7650, .T. ) ;
#5205=FACE_OUTER_BOUND ( 'NONE', #6862, .T. ) ;
#5221=CARTESIAN_POINT ( 'NONE',  ( 44.99999999999992895, -500.0000000000000000, -45.00000000000000711 ) ) ;
#5222=ORIENTED_EDGE ( 'NONE', *, *, #7748, .T. ) ;
#5232=EDGE_LOOP ( 'NONE', ( #7674, #7645, #3603, #1129 ) ) ;
#5241=EDGE_CURVE ( 'NONE', #8027, #5503, #3755, .T. ) ;
#5244=ORIENTED_EDGE ( 'NONE', *, *, #1872, .T. ) ;
#5253=CARTESIAN_POINT ( 'NONE',  ( 0.000000000000000000, 60.00000000000000000, -50.00000000000000000 ) ) ;
#5277=AXIS2_PLACEMENT_3D ( 'NONE', #3320, #5958, #5287 ) ;
#5281=AXIS2_PLACEMENT_3D ( 'NONE', #6900, #3499, #8247 ) ;
#5287=DIRECTION ( 'NONE',  ( 1.000000000000000000, 0.000000000000000000, 0.000000000000000000 ) ) ;
#5291=PLANE ( 'NONE',  #1984 ) ;
#5336=EDGE_LOOP ( 'NONE', ( #3452, #2773, #4460, #5646 ) ) ;
#5364=LINE ( 'NONE', #2099, #4805 ) ;
#5370=ORIENTED_EDGE ( 'NONE', *, *, #643, .F. ) ;
#5381=ORIENTED_EDGE ( 'NONE', *, *, #5147, .F. ) ;
#5392=( LENGTH_UNIT ( ) NAMED_UNIT ( * ) SI_UNIT ( .MILLI., .METRE. ) );
#5406=DIRECTION ( 'NONE',  ( 1.000000000000000000, 0.000000000000000000, 0.000000000000000000 ) ) ;
#5428=EDGE_CURVE ( 'NONE', #6245, #5503, #4954, .T. ) ;
#5433=CARTESIAN_POINT ( 'NONE',  ( 50.00000000000004263, 500.0000000000000000, 50.00000000000000000 ) ) ;
#5438=FACE_OUTER_BOUND ( 'NONE', #3350, .T. ) ;
#5459=ORIENTED_EDGE ( 'NONE', *, *, #7240, .F. ) ;
#5466=CARTESIAN_POINT ( 'NONE',  ( 0.000000000000000000, 60.00000000000000000, -45.00000000000000711 ) ) ;
#5489=CIRCLE ( 'NONE', #4226, 5.499999999999999112 ) ;
#5491=EDGE_CURVE ( 'NONE', #3875, #7175, #4511, .T. ) ;
#5492=DIRECTION ( 'NONE',  ( 0.000000000000000000, 0.000000000000000000, 1.000000000000000000 ) ) ;
#5493=EDGE_CURVE ( 'NONE', #1514, #6221, #7862, .T. ) ;
#5500=DIRECTION ( 'NONE',  ( -0.000000000000000000, -1.000000000000000000, -0.000000000000000000 ) ) ;
#5503=VERTEX_POINT ( 'NONE', #3284 ) ;
#5533=DIRECTION ( 'NONE',  ( 0.000000000000000000, -0.000000000000000000, 1.000000000000000000 ) ) ;
#5547=DIRECTION ( 'NONE',  ( 1.000000000000000000, 0.000000000000000000, 0.000000000000000000 ) ) ;
#5572=ORIENTED_EDGE ( 'NONE', *, *, #2058, .F. ) ;
#5576=VECTOR ( 'NONE', #317, 1000.000000000000000 ) ;
#5594=CARTESIAN_POINT ( 'NONE',  ( -5.500000000000000000, 6.735557395310442023E-16, -50.00000000000000000 ) ) ;
#5599=CARTESIAN_POINT ( 'NONE',  ( -50.00000000000004263, -425.0000000000000000, 3.469446951953614189E-15 ) ) ;
#5602=DIRECTION ( 'NONE',  ( 0.000000000000000000, -0.000000000000000000, 1.000000000000000000 ) ) ;
#5606=FACE_OUTER_BOUND ( 'NONE', #766, .T. ) ;
#5621=DIRECTION ( 'NONE',  ( -0.000000000000000000, -1.000000000000000000, -0.000000000000000000 ) ) ;
#5635=CARTESIAN_POINT ( 'NONE',  ( -50.00000000000004263, 500.0000000000000000, -50.00000000000000000 ) ) ;
#5646=ORIENTED_EDGE ( 'NONE', *, *, #2840, .F. ) ;
#5652=EDGE_CURVE ( 'NONE', #988, #7562, #4699, .T. ) ;
#5669=ORIENTED_EDGE ( 'NONE', *, *, #4427, .T. ) ;
#5675=CARTESIAN_POINT ( 'NONE',  ( -44.99999999999992895, 425.0000000000000000, 25.00000000000001066 ) ) ;
#5678=ADVANCED_FACE ( 'NONE', ( #8480, #7825, #729 ), #3860, .T. ) ;
#5682=LINE ( 'NONE', #6326, #6971 ) ;
#5683=ORIENTED_EDGE ( 'NONE', *, *, #4152, .F. ) ;
#5696=LINE ( 'NONE', #6099, #724 ) ;
#5698=VERTEX_POINT ( 'NONE', #4863 ) ;
#5751=CARTESIAN_POINT ( 'NONE',  ( -44.99999999999992895, -500.0000000000000000, 45.00000000000000711 ) ) ;
#5758=FACE_BOUND ( 'NONE', #7458, .T. ) ;
#5762=LINE ( 'NONE', #430, #7811 ) ;
#5767=AXIS2_PLACEMENT_3D ( 'NONE', #1717, #6394, #423 ) ;
#5769=VERTEX_POINT ( 'NONE', #3532 ) ;
#5772=EDGE_CURVE ( 'NONE', #4565, #8027, #3579, .T. ) ;
#5775=CIRCLE ( 'NONE', #4221, 25.00000000000000711 ) ;
#5776=VERTEX_POINT ( 'NONE', #1906 ) ;
#5781=CARTESIAN_POINT ( 'NONE',  ( 5.499999999999999112, 60.00000000000000000, 50.00000000000000000 ) ) ;
#5795=EDGE_LOOP ( 'NONE', ( #1011, #5370 ) ) ;
#5831=ORIENTED_EDGE ( 'NONE', *, *, #8057, .T. ) ;
#5838=VERTEX_POINT ( 'NONE', #5675 ) ;
#5850=CARTESIAN_POINT ( 'NONE',  ( -50.00000000000004263, 425.0000000000000000, 3.469446951953614189E-15 ) ) ;
#5867=VERTEX_POINT ( 'NONE', #1673 ) ;
#5870=CIRCLE ( 'NONE', #5136, 5.499999999999999112 ) ;
#5873=EDGE_CURVE ( 'NONE', #2950, #1229, #2232, .T. ) ;
#5889=EDGE_CURVE ( 'NONE', #6735, #6221, #5111, .T. ) ;
#5912=CYLINDRICAL_SURFACE ( 'NONE', #7689, 5.500000000000000000 ) ;
#5920=VERTEX_POINT ( 'NONE', #6433 ) ;
#5941=ORIENTED_EDGE ( 'NONE', *, *, #5873, .F. ) ;
#5943=DIRECTION ( 'NONE',  ( -0.000000000000000000, -0.000000000000000000, 1.000000000000000000 ) ) ;
#5958=DIRECTION ( 'NONE',  ( 0.000000000000000000, -0.000000000000000000, 1.000000000000000000 ) ) ;
#5981=ORIENTED_EDGE ( 'NONE', *, *, #5428, .F. ) ;
#5987=DIRECTION ( 'NONE',  ( 1.000000000000000000, 0.000000000000000000, 0.000000000000000000 ) ) ;
#6010=ADVANCED_FACE ( 'NONE', ( #3282 ), #3245, .F. ) ;
#6045=ORIENTED_EDGE ( 'NONE', *, *, #6867, .F. ) ;
#6046=LINE ( 'NONE', #7848, #1113 ) ;
#6053=ORIENTED_EDGE ( 'NONE', *, *, #4982, .F. ) ;
#6055=LINE ( 'NONE', #4548, #876 ) ;
#6058=DIRECTION ( 'NONE',  ( 0.000000000000000000, 0.000000000000000000, 1.000000000000000000 ) ) ;
#6071=EDGE_LOOP ( 'NONE', ( #1048, #7437 ) ) ;
#6079=PLANE ( 'NONE',  #5183 ) ;
#6084=VECTOR ( 'NONE', #7253, 1000.000000000000000 ) ;
#6099=CARTESIAN_POINT ( 'NONE',  ( 50.00000000000004263, -500.0000000000000000, 45.00000000000000711 ) ) ;
#6102=FACE_OUTER_BOUND ( 'NONE', #4963, .T. ) ;
#6110=CARTESIAN_POINT ( 'NONE',  ( -50.00000000000004263, -425.0000000000000000, -25.00000000000000355 ) ) ;
#6114=DIRECTION ( 'NONE',  ( -1.000000000000000000, 0.000000000000000000, 6.938893903907228378E-17 ) ) ;
#6116=DIRECTION ( 'NONE',  ( -1.000000000000000000, 0.000000000000000000, 6.938893903907228378E-17 ) ) ;
#6126=DIRECTION ( 'NONE',  ( -0.000000000000000000, -0.000000000000000000, 1.000000000000000000 ) ) ;
#6130=FACE_OUTER_BOUND ( 'NONE', #5232, .T. ) ;
#6144=DIRECTION ( 'NONE',  ( 0.000000000000000000, -0.000000000000000000, 1.000000000000000000 ) ) ;
#6160=CARTESIAN_POINT ( 'NONE',  ( -44.99999999999992895, 500.0000000000000000, 45.00000000000000711 ) ) ;
#6162=FACE_BOUND ( 'NONE', #6720, .T. ) ;
#6163=ORIENTED_EDGE ( 'NONE', *, *, #1342, .F. ) ;
#6168=DIRECTION ( 'NONE',  ( 0.000000000000000000, 0.000000000000000000, 1.000000000000000000 ) ) ;
#6172=DIRECTION ( 'NONE',  ( 0.000000000000000000, 0.000000000000000000, 1.000000000000000000 ) ) ;
#6182=ORIENTED_EDGE ( 'NONE', *, *, #2437, .T. ) ;
#6193=VECTOR ( 'NONE', #4647, 1000.000000000000000 ) ;
#6200=EDGE_LOOP ( 'NONE', ( #3639, #2632, #7173, #6299 ) ) ;
#6201=EDGE_CURVE ( 'NONE', #748, #7562, #5696, .T. ) ;
#6203=DIRECTION ( 'NONE',  ( 1.000000000000000000, -0.000000000000000000, -6.938893903907228378E-17 ) ) ;
#6206=ORIENTED_EDGE ( 'NONE', *, *, #1342, .T. ) ;
#6207=DIRECTION ( 'NONE',  ( -1.000000000000000000, 0.000000000000000000, -6.938893903907228378E-17 ) ) ;
#6211=ADVANCED_FACE ( 'NONE', ( #7025, #95, #263 ), #6297, .F. ) ;
#6212=CARTESIAN_POINT ( 'NONE',  ( 44.99999999999992895, -425.0000000000000000, -25.00000000000001066 ) ) ;
#6221=VERTEX_POINT ( 'NONE', #8087 ) ;
#6235=VECTOR ( 'NONE', #7599, 1000.000000000000000 ) ;
#6241=DIRECTION ( 'NONE',  ( -0.000000000000000000, -0.000000000000000000, 1.000000000000000000 ) ) ;
#6245=VERTEX_POINT ( 'NONE', #360 ) ;
#6249=DIRECTION ( 'NONE',  ( 0.000000000000000000, 0.000000000000000000, -1.000000000000000000 ) ) ;
#6255=DIRECTION ( 'NONE',  ( 1.000000000000000000, 0.000000000000000000, 0.000000000000000000 ) ) ;
#6259=CARTESIAN_POINT ( 'NONE',  ( 0.000000000000000000, 60.00000000000000000, -50.00000000000000000 ) ) ;
#6272=ADVANCED_FACE ( 'NONE', ( #4406 ), #5912, .F. ) ;
#6274=LINE ( 'NONE', #2251, #1639 ) ;
#6278=CIRCLE ( 'NONE', #2500, 5.500000000000000000 ) ;
#6292=ORIENTED_EDGE ( 'NONE', *, *, #8231, .T. ) ;
#6297=PLANE ( 'NONE',  #6712 ) ;
#6299=ORIENTED_EDGE ( 'NONE', *, *, #5493, .T. ) ;
#6303=VERTEX_POINT ( 'NONE', #8493 ) ;
#6326=CARTESIAN_POINT ( 'NONE',  ( 50.00000000000004263, 500.0000000000000000, 50.00000000000000000 ) ) ;
#6330=VECTOR ( 'NONE', #8553, 1000.000000000000000 ) ;
#6369=ORIENTED_EDGE ( 'NONE', *, *, #8279, .T. ) ;
#6394=DIRECTION ( 'NONE',  ( 1.000000000000000000, -0.000000000000000000, -6.938893903907228378E-17 ) ) ;
#6398=DIRECTION ( 'NONE',  ( 0.000000000000000000, 0.000000000000000000, 1.000000000000000000 ) ) ;
#6402=ORIENTED_EDGE ( 'NONE', *, *, #7889, .F. ) ;
#6409=ORIENTED_EDGE ( 'NONE', *, *, #1759, .F. ) ;
#6411=VECTOR ( 'NONE', #1022, 1000.000000000000000 ) ;
#6433=CARTESIAN_POINT ( 'NONE',  ( -44.99999999999992895, 425.0000000000000000, -25.00000000000000355 ) ) ;
#6438=DIRECTION ( 'NONE',  ( 0.000000000000000000, 0.000000000000000000, 1.000000000000000000 ) ) ;
#6439=VERTEX_POINT ( 'NONE', #7359 ) ;
#6443=AXIS2_PLACEMENT_3D ( 'NONE', #4175, #163, #8105 ) ;
#6455=ORIENTED_EDGE ( 'NONE', *, *, #4427, .F. ) ;
#6462=ORIENTED_EDGE ( 'NONE', *, *, #6539, .T. ) ;
#6470=ADVANCED_FACE ( 'NONE', ( #4624, #6162, #747 ), #6079, .T. ) ;
#6471=AXIS2_PLACEMENT_3D ( 'NONE', #8362, #1203, #3861 ) ;
#6473=DIRECTION ( 'NONE',  ( 0.000000000000000000, 0.000000000000000000, -1.000000000000000000 ) ) ;
#6487=EDGE_CURVE ( 'NONE', #1229, #2950, #4777, .T. ) ;
#6489=CARTESIAN_POINT ( 'NONE',  ( 50.00000000000004263, 500.0000000000000000, -45.00000000000000711 ) ) ;
#6503=EDGE_CURVE ( 'NONE', #5776, #982, #5775, .T. ) ;
#6505=ORIENTED_EDGE ( 'NONE', *, *, #643, .T. ) ;
#6507=CARTESIAN_POINT ( 'NONE',  ( -44.99999999999992895, 500.0000000000000000, -45.00000000000000711 ) ) ;
#6509=DIRECTION ( 'NONE',  ( 1.000000000000000000, 0.000000000000000000, 0.000000000000000000 ) ) ;
#6511=CARTESIAN_POINT ( 'NONE',  ( 50.00000000000004263, 500.0000000000000000, 50.00000000000000000 ) ) ;
#6521=ORIENTED_EDGE ( 'NONE', *, *, #7556, .F. ) ;
#6522=LINE ( 'NONE', #7140, #8335 ) ;
#6524=VERTEX_POINT ( 'NONE', #2053 ) ;
#6526=ORIENTED_EDGE ( 'NONE', *, *, #708, .T. ) ;
#6537=CARTESIAN_POINT ( 'NONE',  ( 50.00000000000004263, 500.0000000000000000, -50.00000000000000000 ) ) ;
#6539=EDGE_CURVE ( 'NONE', #3768, #6303, #6768, .T. ) ;
#6564=VECTOR ( 'NONE', #5621, 1000.000000000000000 ) ;
#6572=ORIENTED_EDGE ( 'NONE', *, *, #2155, .T. ) ;
#6575=ORIENTED_EDGE ( 'NONE', *, *, #7969, .T. ) ;
#6613=DIRECTION ( 'NONE',  ( -1.000000000000000000, 0.000000000000000000, -6.938893903907228378E-17 ) ) ;
#6626=CARTESIAN_POINT ( 'NONE',  ( 0.000000000000000000, 60.00000000000000000, -45.00000000000000711 ) ) ;
#6630=VERTEX_POINT ( 'NONE', #5594 ) ;
#6633=AXIS2_PLACEMENT_3D ( 'NONE', #720, #6058, #4601 ) ;
#6644=EDGE_CURVE ( 'NONE', #5838, #5920, #2614, .T. ) ;
#6675=EDGE_LOOP ( 'NONE', ( #2745, #8476 ) ) ;
#6676=EDGE_CURVE ( 'NONE', #181, #5920, #4524, .T. ) ;
#6679=AXIS2_PLACEMENT_3D ( 'NONE', #6259, #272, #186 ) ;
#6685=ORIENTED_EDGE ( 'NONE', *, *, #7148, .T. ) ;
#6689=LINE ( 'NONE', #8546, #2393 ) ;
#6690=AXIS2_PLACEMENT_3D ( 'NONE', #2611, #4096, #5406 ) ;
#6691=CARTESIAN_POINT ( 'NONE',  ( 5.500000000000000000, 0.000000000000000000, -50.00000000000000000 ) ) ;
#6698=ORIENTED_EDGE ( 'NONE', *, *, #5491, .T. ) ;
#6704=CARTESIAN_POINT ( 'NONE',  ( -5.500000000000000000, 6.735557395310442023E-16, -50.00000000000000000 ) ) ;
#6712=AXIS2_PLACEMENT_3D ( 'NONE', #5433, #2927, #2398 ) ;
#6714=CARTESIAN_POINT ( 'NONE',  ( 50.00000000000004263, 500.0000000000000000, -50.00000000000000000 ) ) ;
#6720=EDGE_LOOP ( 'NONE', ( #3502, #4886 ) ) ;
#6730=VECTOR ( 'NONE', #1761, 1000.000000000000000 ) ;
#6735=VERTEX_POINT ( 'NONE', #5221 ) ;
#6763=DIRECTION ( 'NONE',  ( 6.938893903907228378E-17, 0.000000000000000000, -1.000000000000000000 ) ) ;
#6768=LINE ( 'NONE', #6893, #8198 ) ;
#6775=LINE ( 'NONE', #3458, #1852 ) ;
#6800=DIRECTION ( 'NONE',  ( 1.000000000000000000, 0.000000000000000000, -6.938893903907228378E-17 ) ) ;
#6813=AXIS2_PLACEMENT_3D ( 'NONE', #41, #711, #2539 ) ;
#6819=EDGE_CURVE ( 'NONE', #6524, #5867, #6522, .T. ) ;
#6824=DIRECTION ( 'NONE',  ( 6.938893903907228378E-17, 0.000000000000000000, -1.000000000000000000 ) ) ;
#6835=CARTESIAN_POINT ( 'NONE',  ( 50.00000000000004263, -425.0000000000000000, -3.469446951953614189E-15 ) ) ;
#6836=ADVANCED_FACE ( 'NONE', ( #1954, #4090, #4749 ), #8010, .T. ) ;
#6862=EDGE_LOOP ( 'NONE', ( #675, #2001, #3274, #1901 ) ) ;
#6867=EDGE_CURVE ( 'NONE', #4067, #6439, #2742, .T. ) ;
#6869=CARTESIAN_POINT ( 'NONE',  ( 0.000000000000000000, 0.000000000000000000, 50.00000000000000000 ) ) ;
#6875=ORIENTED_EDGE ( 'NONE', *, *, #5493, .F. ) ;
#6886=ORIENTED_EDGE ( 'NONE', *, *, #4663, .F. ) ;
#6893=CARTESIAN_POINT ( 'NONE',  ( 44.99999999999992895, 500.0000000000000000, 50.00000000000000000 ) ) ;
#6894=ORIENTED_EDGE ( 'NONE', *, *, #1872, .F. ) ;
#6900=CARTESIAN_POINT ( 'NONE',  ( -50.00000000000004263, 425.0000000000000000, 3.469446951953614189E-15 ) ) ;
#6929=ORIENTED_EDGE ( 'NONE', *, *, #1759, .T. ) ;
#6940=DIRECTION ( 'NONE',  ( -1.000000000000000000, 0.000000000000000000, 0.000000000000000000 ) ) ;
#6949=DIRECTION ( 'NONE',  ( -1.000000000000000000, 0.000000000000000000, -6.938893903907228378E-17 ) ) ;
#6967=LINE ( 'NONE', #1510, #2026 ) ;
#6971=VECTOR ( 'NONE', #7699, 1000.000000000000000 ) ;
#6989=ORIENTED_EDGE ( 'NONE', *, *, #3587, .F. ) ;
#6994=CYLINDRICAL_SURFACE ( 'NONE', #6679, 5.499999999999999112 ) ;
#6995=AXIS2_PLACEMENT_3D ( 'NONE', #7654, #5533, #950 ) ;
#7009=AXIS2_PLACEMENT_3D ( 'NONE', #3652, #5072, #426 ) ;
#7021=EDGE_LOOP ( 'NONE', ( #4882, #2755 ) ) ;
#7025=FACE_BOUND ( 'NONE', #5795, .T. ) ;
#7036=DIRECTION ( 'NONE',  ( -0.000000000000000000, -0.000000000000000000, 1.000000000000000000 ) ) ;
#7046=DIRECTION ( 'NONE',  ( -1.000000000000000000, 0.000000000000000000, -6.938893903907228378E-17 ) ) ;
#7082=CARTESIAN_POINT ( 'NONE',  ( -50.00000000000004263, -425.0000000000000000, -25.00000000000000355 ) ) ;
#7106=AXIS2_PLACEMENT_3D ( 'NONE', #3736, #7046, #6398 ) ;
#7109=DIRECTION ( 'NONE',  ( 0.000000000000000000, -0.000000000000000000, 1.000000000000000000 ) ) ;
#7113=LINE ( 'NONE', #3014, #420 ) ;
#7119=CARTESIAN_POINT ( 'NONE',  ( 5.499999999999999112, 60.00000000000000000, -50.00000000000000000 ) ) ;
#7123=CARTESIAN_POINT ( 'NONE',  ( -5.499999999999999112, 60.00000000000000000, -50.00000000000000000 ) ) ;
#7133=VERTEX_POINT ( 'NONE', #6511 ) ;
#7135=AXIS2_PLACEMENT_3D ( 'NONE', #3814, #791, #2151 ) ;
#7138=FACE_OUTER_BOUND ( 'NONE', #2860, .T. ) ;
#7140=CARTESIAN_POINT ( 'NONE',  ( -50.00000000000004263, 500.0000000000000000, 50.00000000000000000 ) ) ;
#7145=EDGE_CURVE ( 'NONE', #477, #4124, #4298, .T. ) ;
#7146=ORIENTED_EDGE ( 'NONE', *, *, #2924, .T. ) ;
#7148=EDGE_CURVE ( 'NONE', #8288, #450, #2489, .T. ) ;
#7155=EDGE_CURVE ( 'NONE', #4756, #3262, #2082, .T. ) ;
#7173=ORIENTED_EDGE ( 'NONE', *, *, #48, .T. ) ;
#7175=VERTEX_POINT ( 'NONE', #1043 ) ;
#7179=CARTESIAN_POINT ( 'NONE',  ( 50.00000000000004263, 425.0000000000000000, -3.469446951953614189E-15 ) ) ;
#7208=DIRECTION ( 'NONE',  ( 0.000000000000000000, -0.000000000000000000, 1.000000000000000000 ) ) ;
#7240=EDGE_CURVE ( 'NONE', #450, #8288, #7640, .T. ) ;
#7253=DIRECTION ( 'NONE',  ( -0.000000000000000000, -1.000000000000000000, -0.000000000000000000 ) ) ;
#7257=CARTESIAN_POINT ( 'NONE',  ( -44.99999999999992895, -425.0000000000000000, 25.00000000000001066 ) ) ;
#7280=( NAMED_UNIT ( * ) PLANE_ANGLE_UNIT ( ) SI_UNIT ( $, .RADIAN. ) );
#7287=CARTESIAN_POINT ( 'NONE',  ( 50.00000000000004263, -500.0000000000000000, 50.00000000000000000 ) ) ;
#7294=EDGE_LOOP ( 'NONE', ( #6455, #6402 ) ) ;
#7318=CARTESIAN_POINT ( 'NONE',  ( -5.499999999999999112, 60.00000000000000000, 50.00000000000000000 ) ) ;
#7328=ORIENTED_EDGE ( 'NONE', *, *, #8057, .F. ) ;
#7329=DIRECTION ( 'NONE',  ( -1.000000000000000000, 0.000000000000000000, 0.000000000000000000 ) ) ;
#7334=CARTESIAN_POINT ( 'NONE',  ( 5.499999999999999112, 60.00000000000000000, -50.00000000000000000 ) ) ;
#7345=CARTESIAN_POINT ( 'NONE',  ( -44.99999999999992895, 500.0000000000000000, 45.00000000000000711 ) ) ;
#7356=DIRECTION ( 'NONE',  ( -1.000000000000000000, 0.000000000000000000, 0.000000000000000000 ) ) ;
#7359=CARTESIAN_POINT ( 'NONE',  ( -5.500000000000000000, 6.735557395310442023E-16, 50.00000000000000000 ) ) ;
#7387=CYLINDRICAL_SURFACE ( 'NONE', #3802, 5.499999999999999112 ) ;
#7420=DIRECTION ( 'NONE',  ( 1.000000000000000000, 0.000000000000000000, 0.000000000000000000 ) ) ;
#7437=ORIENTED_EDGE ( 'NONE', *, *, #7155, .F. ) ;
#7438=CARTESIAN_POINT ( 'NONE',  ( 50.00000000000004263, 500.0000000000000000, -50.00000000000000000 ) ) ;
#7445=VECTOR ( 'NONE', #3440, 1000.000000000000000 ) ;
#7449=CARTESIAN_POINT ( 'NONE',  ( -50.00000000000004263, 425.0000000000000000, 3.469446951953614189E-15 ) ) ;
#7454=CARTESIAN_POINT ( 'NONE',  ( 0.000000000000000000, 0.000000000000000000, -50.00000000000000000 ) ) ;
#7458=EDGE_LOOP ( 'NONE', ( #1845, #415 ) ) ;
#7463=CYLINDRICAL_SURFACE ( 'NONE', #7695, 25.00000000000000711 ) ;
#7469=CIRCLE ( 'NONE', #6633, 5.499999999999999112 ) ;
#7478=DIRECTION ( 'NONE',  ( 0.000000000000000000, 0.000000000000000000, 1.000000000000000000 ) ) ;
#7479=EDGE_LOOP ( 'NONE', ( #715, #3810 ) ) ;
#7493=CARTESIAN_POINT ( 'NONE',  ( 44.99999999999992895, 500.0000000000000000, 50.00000000000000000 ) ) ;
#7495=ORIENTED_EDGE ( 'NONE', *, *, #2058, .T. ) ;
#7501=AXIS2_PLACEMENT_3D ( 'NONE', #8395, #1812, #6473 ) ;
#7510=DIRECTION ( 'NONE',  ( 0.000000000000000000, 0.000000000000000000, 1.000000000000000000 ) ) ;
#7525=ORIENTED_EDGE ( 'NONE', *, *, #5428, .T. ) ;
#7538=ORIENTED_EDGE ( 'NONE', *, *, #4056, .F. ) ;
#7547=ORIENTED_EDGE ( 'NONE', *, *, #708, .F. ) ;
#7552=DIRECTION ( 'NONE',  ( 0.000000000000000000, 0.000000000000000000, -1.000000000000000000 ) ) ;
#7555=CARTESIAN_POINT ( 'NONE',  ( 5.499999999999999112, 60.00000000000000000, 45.00000000000000000 ) ) ;
#7556=EDGE_CURVE ( 'NONE', #5769, #4067, #8479, .T. ) ;
#7562=VERTEX_POINT ( 'NONE', #5751 ) ;
#7563=AXIS2_PLACEMENT_3D ( 'NONE', #4203, #7478, #3512 ) ;
#7574=ORIENTED_EDGE ( 'NONE', *, *, #7748, .F. ) ;
#7588=VECTOR ( 'NONE', #1238, 1000.000000000000000 ) ;
#7594=CIRCLE ( 'NONE', #4947, 25.00000000000000711 ) ;
#7599=DIRECTION ( 'NONE',  ( 6.938893903907228378E-17, 0.000000000000000000, -1.000000000000000000 ) ) ;
#7602=AXIS2_PLACEMENT_3D ( 'NONE', #1862, #6613, #3954 ) ;
#7635=CIRCLE ( 'NONE', #829, 25.00000000000000711 ) ;
#7640=CIRCLE ( 'NONE', #2913, 25.00000000000000711 ) ;
#7645=ORIENTED_EDGE ( 'NONE', *, *, #5204, .F. ) ;
#7650=CIRCLE ( 'NONE', #5130, 25.00000000000000711 ) ;
#7654=CARTESIAN_POINT ( 'NONE',  ( 0.000000000000000000, 60.00000000000000000, 45.00000000000000000 ) ) ;
#7674=ORIENTED_EDGE ( 'NONE', *, *, #8558, .F. ) ;
#7686=ORIENTED_EDGE ( 'NONE', *, *, #7148, .F. ) ;
#7689=AXIS2_PLACEMENT_3D ( 'NONE', #1740, #3267, #615 ) ;
#7695=AXIS2_PLACEMENT_3D ( 'NONE', #3588, #4885, #6249 ) ;
#7699=DIRECTION ( 'NONE',  ( -1.000000000000000000, 0.000000000000000000, 0.000000000000000000 ) ) ;
#7704=DIRECTION ( 'NONE',  ( 1.000000000000000000, 0.000000000000000000, -6.938893903907228378E-17 ) ) ;
#7739=EDGE_LOOP ( 'NONE', ( #5572, #2242 ) ) ;
#7748=EDGE_CURVE ( 'NONE', #3548, #4837, #6046, .T. ) ;
#7750=UNCERTAINTY_MEASURE_WITH_UNIT (LENGTH_MEASURE( 1.000000000000000082E-05 ), #7929, 'distance_accuracy_value', 'NONE');
#7762=LINE ( 'NONE', #7119, #1944 ) ;
#7770=DIRECTION ( 'NONE',  ( -1.000000000000000000, 0.000000000000000000, 0.000000000000000000 ) ) ;
#7774=CARTESIAN_POINT ( 'NONE',  ( -50.00000000000004263, -425.0000000000000000, 25.00000000000001066 ) ) ;
#7779=EDGE_LOOP ( 'NONE', ( #4616, #2876, #8570, #7146 ) ) ;
#7792=ORIENTED_EDGE ( 'NONE', *, *, #1216, .T. ) ;
#7797=EDGE_LOOP ( 'NONE', ( #2907, #4245, #4994, #7574 ) ) ;
#7811=VECTOR ( 'NONE', #5034, 1000.000000000000000 ) ;
#7825=FACE_BOUND ( 'NONE', #2004, .T. ) ;
#7848=CARTESIAN_POINT ( 'NONE',  ( 50.00000000000004263, -500.0000000000000000, -50.00000000000000000 ) ) ;
#7862=LINE ( 'NONE', #636, #6084 ) ;
#7865=ADVANCED_FACE ( 'NONE', ( #7987, #2016, #4278 ), #4240, .F. ) ;
#7879=ADVANCED_FACE ( 'NONE', ( #6130 ), #2231, .F. ) ;
#7889=EDGE_CURVE ( 'NONE', #7175, #2167, #5870, .T. ) ;
#7892=PRODUCT_DEFINITION ( 'UNKNOWN', '', #3119, #2373 ) ;
#7909=CYLINDRICAL_SURFACE ( 'NONE', #4593, 25.00000000000000711 ) ;
#7923=VECTOR ( 'NONE', #8422, 1000.000000000000000 ) ;
#7926=CLOSED_SHELL ( 'NONE', ( #5166, #3225, #8580, #2071, #4588, #1110, #52, #8568, #4454, #3497, #6211, #7865, #5678, #6470, #3244, #6836, #696, #1672, #7879, #4728, #5120, #3920, #6272, #4925, #6010, #4410 ) ) ;
#7929=( LENGTH_UNIT ( ) NAMED_UNIT ( * ) SI_UNIT ( .MILLI., .METRE. ) );
#7930=ORIENTED_EDGE ( 'NONE', *, *, #6201, .F. ) ;
#7946=LINE ( 'NONE', #1978, #6193 ) ;
#7968=ORIENTED_EDGE ( 'NONE', *, *, #7889, .T. ) ;
#7969=EDGE_CURVE ( 'NONE', #6439, #3947, #6278, .T. ) ;
#7981=AXIS2_PLACEMENT_3D ( 'NONE', #8090, #816, #3428 ) ;
#7987=FACE_BOUND ( 'NONE', #512, .T. ) ;
#8010=PLANE ( 'NONE',  #1512 ) ;
#8012=ORIENTED_EDGE ( 'NONE', *, *, #1993, .F. ) ;
#8019=LINE ( 'NONE', #2049, #8126 ) ;
#8021=DIRECTION ( 'NONE',  ( -0.000000000000000000, -1.000000000000000000, -0.000000000000000000 ) ) ;
#8027=VERTEX_POINT ( 'NONE', #1785 ) ;
#8031=ORIENTED_EDGE ( 'NONE', *, *, #2250, .F. ) ;
#8054=FACE_BOUND ( 'NONE', #3908, .T. ) ;
#8056=DIRECTION ( 'NONE',  ( 1.000000000000000000, -0.000000000000000000, -6.938893903907228378E-17 ) ) ;
#8057=EDGE_CURVE ( 'NONE', #748, #6735, #5138, .T. ) ;
#8066=CIRCLE ( 'NONE', #5277, 5.500000000000000000 ) ;
#8076=VECTOR ( 'NONE', #6203, 1000.000000000000000 ) ;
#8087=CARTESIAN_POINT ( 'NONE',  ( -44.99999999999992895, -500.0000000000000000, -45.00000000000000711 ) ) ;
#8090=CARTESIAN_POINT ( 'NONE',  ( -50.00000000000004263, 425.0000000000000000, 3.469446951953614189E-15 ) ) ;
#8102=ORIENTED_EDGE ( 'NONE', *, *, #4982, .T. ) ;
#8105=DIRECTION ( 'NONE',  ( 0.000000000000000000, 0.000000000000000000, 1.000000000000000000 ) ) ;
#8126=VECTOR ( 'NONE', #7356, 1000.000000000000000 ) ;
#8128=CARTESIAN_POINT ( 'NONE',  ( -44.99999999999992895, 500.0000000000000000, 50.00000000000000000 ) ) ;
#8129=EDGE_LOOP ( 'NONE', ( #4835, #5024, #915, #5244 ) ) ;
#8145=EDGE_LOOP ( 'NONE', ( #5199, #6409 ) ) ;
#8165=CARTESIAN_POINT ( 'NONE',  ( 50.00000000000004263, -425.0000000000000000, -3.469446951953614189E-15 ) ) ;
#8183=CYLINDRICAL_SURFACE ( 'NONE', #4202, 5.500000000000000000 ) ;
#8198=VECTOR ( 'NONE', #2222, 1000.000000000000000 ) ;
#8206=AXIS2_PLACEMENT_3D ( 'NONE', #1655, #6949, #8333 ) ;
#8223=VECTOR ( 'NONE', #7770, 1000.000000000000000 ) ;
#8231=EDGE_CURVE ( 'NONE', #8316, #181, #201, .T. ) ;
#8247=DIRECTION ( 'NONE',  ( 0.000000000000000000, 0.000000000000000000, -1.000000000000000000 ) ) ;
#8279=EDGE_CURVE ( 'NONE', #4655, #982, #2744, .T. ) ;
#8281=CARTESIAN_POINT ( 'NONE',  ( -44.99999999999992895, 425.0000000000000000, 3.122502256758253953E-15 ) ) ;
#8287=DIRECTION ( 'NONE',  ( 1.000000000000000000, 0.000000000000000000, 0.000000000000000000 ) ) ;
#8288=VERTEX_POINT ( 'NONE', #6110 ) ;
#8301=VECTOR ( 'NONE', #1340, 1000.000000000000000 ) ;
#8303=ORIENTED_EDGE ( 'NONE', *, *, #4501, .T. ) ;
#8316=VERTEX_POINT ( 'NONE', #206 ) ;
#8328=DIRECTION ( 'NONE',  ( -6.938893903907228378E-17, 0.000000000000000000, -1.000000000000000000 ) ) ;
#8333=DIRECTION ( 'NONE',  ( 0.000000000000000000, 0.000000000000000000, 1.000000000000000000 ) ) ;
#8335=VECTOR ( 'NONE', #1166, 1000.000000000000000 ) ;
#8342=DIRECTION ( 'NONE',  ( 1.000000000000000000, 0.000000000000000000, 0.000000000000000000 ) ) ;
#8362=CARTESIAN_POINT ( 'NONE',  ( -50.00000000000004263, 425.0000000000000000, 3.469446951953614189E-15 ) ) ;
#8367=EDGE_CURVE ( 'NONE', #1742, #6630, #750, .T. ) ;
#8380=ORIENTED_EDGE ( 'NONE', *, *, #7240, .T. ) ;
#8388=FACE_BOUND ( 'NONE', #7021, .T. ) ;
#8395=CARTESIAN_POINT ( 'NONE',  ( -50.00000000000004263, -425.0000000000000000, 3.469446951953614189E-15 ) ) ;
#8396=AXIS2_PLACEMENT_3D ( 'NONE', #179, #6168, #5547 ) ;
#8406=DIRECTION ( 'NONE',  ( 1.000000000000000000, -0.000000000000000000, -6.938893903907228378E-17 ) ) ;
#8411=EDGE_CURVE ( 'NONE', #4726, #4794, #5489, .T. ) ;
#8412=FACE_OUTER_BOUND ( 'NONE', #5186, .T. ) ;
#8422=DIRECTION ( 'NONE',  ( -0.000000000000000000, -0.000000000000000000, 1.000000000000000000 ) ) ;
#8428=ORIENTED_EDGE ( 'NONE', *, *, #4418, .F. ) ;
#8430=ORIENTED_EDGE ( 'NONE', *, *, #1747, .T. ) ;
#8439=ORIENTED_EDGE ( 'NONE', *, *, #7145, .T. ) ;
#8440=ORIENTED_EDGE ( 'NONE', *, *, #1046, .F. ) ;
#8454=LINE ( 'NONE', #1745, #7923 ) ;
#8457=CARTESIAN_POINT ( 'NONE',  ( 44.99999999999992895, 425.0000000000000000, -3.122502256758253953E-15 ) ) ;
#8459=AXIS2_PLACEMENT_3D ( 'NONE', #4977, #7036, #3724 ) ;
#8465=CARTESIAN_POINT ( 'NONE',  ( 44.99999999999992895, 425.0000000000000000, -25.00000000000001066 ) ) ;
#8473=CARTESIAN_POINT ( 'NONE',  ( 0.000000000000000000, 60.00000000000000000, 50.00000000000000000 ) ) ;
#8476=ORIENTED_EDGE ( 'NONE', *, *, #2250, .T. ) ;
#8477=DIRECTION ( 'NONE',  ( 1.000000000000000000, -0.000000000000000000, -6.938893903907228378E-17 ) ) ;
#8479=CIRCLE ( 'NONE', #4237, 5.500000000000000000 ) ;
#8480=FACE_BOUND ( 'NONE', #8523, .T. ) ;
#8485=AXIS2_PLACEMENT_3D ( 'NONE', #4929, #7109, #8287 ) ;
#8493=CARTESIAN_POINT ( 'NONE',  ( 44.99999999999992895, 500.0000000000000000, -45.00000000000000711 ) ) ;
#8511=DIRECTION ( 'NONE',  ( 0.000000000000000000, -0.000000000000000000, 1.000000000000000000 ) ) ;
#8516=FACE_OUTER_BOUND ( 'NONE', #1826, .T. ) ;
#8523=EDGE_LOOP ( 'NONE', ( #6685, #8380 ) ) ;
#8528=CIRCLE ( 'NONE', #4087, 5.499999999999999112 ) ;
#8531=EDGE_LOOP ( 'NONE', ( #3258, #560 ) ) ;
#8537=LINE ( 'NONE', #6537, #880 ) ;
#8546=CARTESIAN_POINT ( 'NONE',  ( -50.00000000000004263, 500.0000000000000000, 50.00000000000000000 ) ) ;
#8553=DIRECTION ( 'NONE',  ( 1.000000000000000000, -0.000000000000000000, -6.938893903907228378E-17 ) ) ;
#8558=EDGE_CURVE ( 'NONE', #8316, #5838, #1466, .T. ) ;
#8568=ADVANCED_FACE ( 'NONE', ( #5438 ), #4782, .F. ) ;
#8570=ORIENTED_EDGE ( 'NONE', *, *, #3994, .T. ) ;
#8575=AXIS2_PLACEMENT_3D ( 'NONE', #3448, #6116, #2833 ) ;
#8577=FACE_OUTER_BOUND ( 'NONE', #127, .T. ) ;
#8580=ADVANCED_FACE ( 'NONE', ( #6102 ), #7387, .F. ) ;
#8581=APPLICATION_CONTEXT ( 'automotive_design' ) ;
#8587=AXIS2_PLACEMENT_3D ( 'NONE', #8281, #6207, #1522 ) ;
#8671=COLOUR_RGB('Off White',0.89,0.88,0.83);
#8672=FILL_AREA_STYLE_COLOUR('',#8671);
#8673=FILL_AREA_STYLE('',(#8672));
#8674=SURFACE_STYLE_FILL_AREA(#8673);
#8675=SURFACE_SIDE_STYLE('',(#8674));
#8676=SURFACE_STYLE_USAGE(.BOTH.,#8675);
#8677=PRESENTATION_STYLE_ASSIGNMENT((#8676));
ENDSEC;
END-ISO-10303-21;
